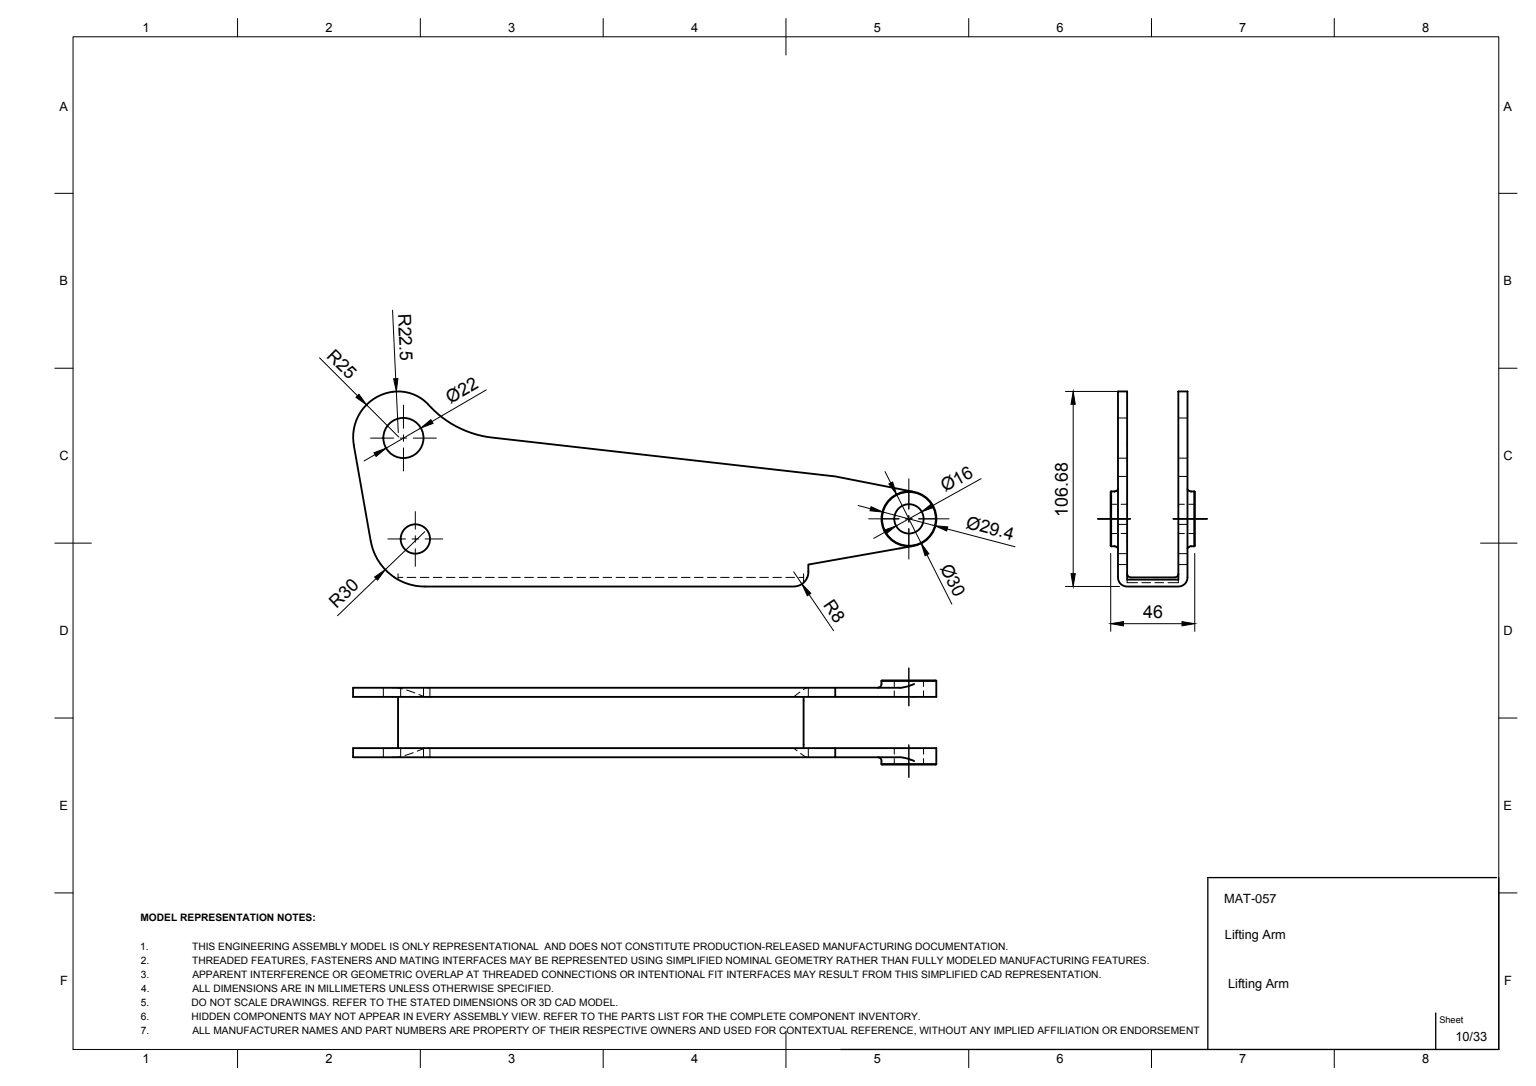
ISO-10303-21;
HEADER;
/* Generated by software containing ST-Developer
 * from STEP Tools, Inc. (www.steptools.com) 
 */

FILE_DESCRIPTION(
/* description */ ('STEP AP214', 'CAx-IF Rec.Pracs.---Representation and Presentation of Product Manufa
cturing Information (PMI)---4.0---2014-10-13'),
/* implementation_level */ '2;1');

FILE_NAME(
/* name */ 'Lifting Arm.step',
/* time_stamp */ '2026-10-28T23:34:22+01:00',
/* author */ (''),
/* organization */ (''),
/* preprocessor_version */ 'ST-DEVELOPER v20.2',
/* originating_system */ 'Autodesk Translation Framework v15.17.0.0',
/* authorisation */ '');

FILE_SCHEMA (('AP242_MANAGED_MODEL_BASED_3D_ENGINEERING_MIM_LF { 1 0 10303 442 2 1 4 }'));
ENDSEC;

DATA;
#10=MECHANICAL_DESIGN_GEOMETRIC_PRESENTATION_REPRESENTATION('',(#251),#27807);
#207=SHAPE_REPRESENTATION_RELATIONSHIP('SRR','None',#27902,#229);
#229=ADVANCED_BREP_SHAPE_REPRESENTATION('',(#280),#27782);
#251=STYLED_ITEM('',(#28070),#280);
#280=MANIFOLD_SOLID_BREP('Body1',#12027);
#363=FACE_BOUND('',#2137,.T.);
#364=FACE_BOUND('',#2138,.T.);
#365=FACE_BOUND('',#2142,.T.);
#366=FACE_BOUND('',#2143,.T.);
#367=FACE_BOUND('',#2144,.T.);
#368=FACE_BOUND('',#2152,.T.);
#369=FACE_BOUND('',#2153,.T.);
#370=FACE_BOUND('',#2178,.T.);
#371=FACE_BOUND('',#2179,.T.);
#372=FACE_BOUND('',#2180,.T.);
#373=FACE_BOUND('',#2182,.T.);
#374=FACE_BOUND('',#2184,.T.);
#514=PLANE('',#12657);
#515=PLANE('',#12665);
#516=PLANE('',#12669);
#517=PLANE('',#12678);
#518=PLANE('',#12681);
#519=PLANE('',#12684);
#520=PLANE('',#12685);
#521=PLANE('',#12686);
#522=PLANE('',#12693);
#523=PLANE('',#12721);
#524=PLANE('',#12726);
#525=PLANE('',#12727);
#526=PLANE('',#12728);
#527=PLANE('',#12729);
#528=PLANE('',#12730);
#529=PLANE('',#12731);
#530=PLANE('',#12732);
#531=PLANE('',#12733);
#532=PLANE('',#12735);
#533=PLANE('',#12736);
#534=PLANE('',#12739);
#535=PLANE('',#12742);
#825=TOROIDAL_SURFACE('',#12701,17.,2.);
#826=TOROIDAL_SURFACE('',#12704,17.,2.);
#866=B_SPLINE_CURVE_WITH_KNOTS('',3,(#18580,#18581,#18582,#18583,#18584,
#18585,#18586,#18587),.UNSPECIFIED.,.F.,.F.,(4,2,2,4),(1.64653183621645,
1.82629619953337,2.00606056285029,2.42476187739513),.UNSPECIFIED.);
#867=B_SPLINE_CURVE_WITH_KNOTS('',3,(#18614,#18615,#18616,#18617),
 .UNSPECIFIED.,.F.,.F.,(4,4),(0.,0.783684993176865),.UNSPECIFIED.);
#868=B_SPLINE_CURVE_WITH_KNOTS('',3,(#18636,#18637,#18638,#18639),
 .UNSPECIFIED.,.F.,.F.,(4,4),(-2.42476187739513,-1.64107688421826),
 .UNSPECIFIED.);
#869=B_SPLINE_CURVE_WITH_KNOTS('',3,(#18646,#18647,#18648,#18649,#18650,
#18651,#18652,#18653),.UNSPECIFIED.,.F.,.F.,(4,2,2,4),(-0.778230041178668,
-0.598465677861747,-0.418701314544826,0.),.UNSPECIFIED.);
#870=B_SPLINE_CURVE_WITH_KNOTS('',3,(#18695,#18696,#18697,#18698,#18699,
#18700,#18701,#18702),.UNSPECIFIED.,.F.,.F.,(4,2,2,4),(3.68263908945476,
4.12349601732247,4.56435294519017,5.44606680092558),.UNSPECIFIED.);
#871=B_SPLINE_CURVE_WITH_KNOTS('',3,(#18705,#18706,#18707,#18708,#18709,
#18710,#18711,#18712,#18713,#18714),.UNSPECIFIED.,.F.,.F.,(4,2,2,2,4),(0.,
0.473183086940068,0.946366173880136,1.33890283846488,1.73143950304963),
 .UNSPECIFIED.);
#872=B_SPLINE_CURVE_WITH_KNOTS('',3,(#18725,#18726,#18727,#18728,#18729,
#18730,#18731,#18732,#18733,#18734),.UNSPECIFIED.,.F.,.F.,(4,2,2,2,4),(0.,
0.287218434472245,0.57443686894449,0.807390418400316,1.04034396785614),
 .UNSPECIFIED.);
#873=B_SPLINE_CURVE_WITH_KNOTS('',3,(#18741,#18742,#18743,#18744,#18745,
#18746,#18747,#18748,#18749,#18750),.UNSPECIFIED.,.F.,.F.,(4,2,2,2,4),(2.56810417568796,
2.77815458546554,2.98820499524312,3.29809009872942,3.60797520221572),
 .UNSPECIFIED.);
#1048=CYLINDRICAL_SURFACE('',#12654,22.5);
#1049=CYLINDRICAL_SURFACE('',#12666,22.5);
#1050=CYLINDRICAL_SURFACE('',#12679,55.);
#1051=CYLINDRICAL_SURFACE('',#12682,55.);
#1052=CYLINDRICAL_SURFACE('',#12707,11.);
#1053=CYLINDRICAL_SURFACE('',#12708,7.99999999999999);
#1054=CYLINDRICAL_SURFACE('',#12709,7.99999999999999);
#1055=CYLINDRICAL_SURFACE('',#12711,15.);
#1056=CYLINDRICAL_SURFACE('',#12713,11.);
#1057=CYLINDRICAL_SURFACE('',#12715,7.99999999999999);
#1058=CYLINDRICAL_SURFACE('',#12717,7.99999999999999);
#1059=CYLINDRICAL_SURFACE('',#12720,15.);
#1060=CYLINDRICAL_SURFACE('',#12722,30.);
#1061=CYLINDRICAL_SURFACE('',#12724,7.99999999999999);
#1062=CYLINDRICAL_SURFACE('',#12737,25.);
#1063=CYLINDRICAL_SURFACE('',#12738,25.);
#1064=CYLINDRICAL_SURFACE('',#12745,5.);
#1065=CYLINDRICAL_SURFACE('',#12746,5.);
#1066=CYLINDRICAL_SURFACE('',#12747,2.);
#1067=CYLINDRICAL_SURFACE('',#12748,2.);
#1410=FACE_OUTER_BOUND('',#2135,.T.);
#1411=FACE_OUTER_BOUND('',#2136,.T.);
#1412=FACE_OUTER_BOUND('',#2139,.T.);
#1413=FACE_OUTER_BOUND('',#2140,.T.);
#1414=FACE_OUTER_BOUND('',#2141,.T.);
#1415=FACE_OUTER_BOUND('',#2145,.T.);
#1416=FACE_OUTER_BOUND('',#2146,.T.);
#1417=FACE_OUTER_BOUND('',#2147,.T.);
#1418=FACE_OUTER_BOUND('',#2148,.T.);
#1419=FACE_OUTER_BOUND('',#2149,.T.);
#1420=FACE_OUTER_BOUND('',#2150,.T.);
#1421=FACE_OUTER_BOUND('',#2151,.T.);
#1422=FACE_OUTER_BOUND('',#2154,.T.);
#1423=FACE_OUTER_BOUND('',#2155,.T.);
#1424=FACE_OUTER_BOUND('',#2156,.T.);
#1425=FACE_OUTER_BOUND('',#2157,.T.);
#1426=FACE_OUTER_BOUND('',#2158,.T.);
#1427=FACE_OUTER_BOUND('',#2159,.T.);
#1428=FACE_OUTER_BOUND('',#2160,.T.);
#1429=FACE_OUTER_BOUND('',#2161,.T.);
#1430=FACE_OUTER_BOUND('',#2162,.T.);
#1431=FACE_OUTER_BOUND('',#2163,.T.);
#1432=FACE_OUTER_BOUND('',#2164,.T.);
#1433=FACE_OUTER_BOUND('',#2165,.T.);
#1434=FACE_OUTER_BOUND('',#2166,.T.);
#1435=FACE_OUTER_BOUND('',#2167,.T.);
#1436=FACE_OUTER_BOUND('',#2168,.T.);
#1437=FACE_OUTER_BOUND('',#2169,.T.);
#1438=FACE_OUTER_BOUND('',#2170,.T.);
#1439=FACE_OUTER_BOUND('',#2171,.T.);
#1440=FACE_OUTER_BOUND('',#2172,.T.);
#1441=FACE_OUTER_BOUND('',#2173,.T.);
#1442=FACE_OUTER_BOUND('',#2174,.T.);
#1443=FACE_OUTER_BOUND('',#2175,.T.);
#1444=FACE_OUTER_BOUND('',#2176,.T.);
#1445=FACE_OUTER_BOUND('',#2177,.T.);
#1446=FACE_OUTER_BOUND('',#2181,.T.);
#1447=FACE_OUTER_BOUND('',#2183,.T.);
#1448=FACE_OUTER_BOUND('',#2185,.T.);
#1449=FACE_OUTER_BOUND('',#2186,.T.);
#1450=FACE_OUTER_BOUND('',#2187,.T.);
#1451=FACE_OUTER_BOUND('',#2188,.T.);
#1452=FACE_OUTER_BOUND('',#2189,.T.);
#1453=FACE_OUTER_BOUND('',#2190,.T.);
#1454=FACE_OUTER_BOUND('',#2191,.T.);
#1455=FACE_OUTER_BOUND('',#2192,.T.);
#2135=EDGE_LOOP('',(#8699,#8700,#8701,#8702));
#2136=EDGE_LOOP('',(#8703,#8704,#8705,#8706,#8707,#8708,#8709,#8710,#8711,
#8712,#8713,#8714,#8715));
#2137=EDGE_LOOP('',(#8716));
#2138=EDGE_LOOP('',(#8717));
#2139=EDGE_LOOP('',(#8718,#8719,#8720,#8721));
#2140=EDGE_LOOP('',(#8722,#8723,#8724,#8725));
#2141=EDGE_LOOP('',(#8726,#8727,#8728,#8729,#8730,#8731,#8732,#8733,#8734,
#8735,#8736,#8737,#8738,#8739,#8740));
#2142=EDGE_LOOP('',(#8741));
#2143=EDGE_LOOP('',(#8742));
#2144=EDGE_LOOP('',(#8743));
#2145=EDGE_LOOP('',(#8744,#8745,#8746,#8747));
#2146=EDGE_LOOP('',(#8748,#8749,#8750,#8751));
#2147=EDGE_LOOP('',(#8752,#8753,#8754,#8755));
#2148=EDGE_LOOP('',(#8756,#8757,#8758,#8759));
#2149=EDGE_LOOP('',(#8760,#8761,#8762,#8763));
#2150=EDGE_LOOP('',(#8764,#8765,#8766,#8767,#8768));
#2151=EDGE_LOOP('',(#8769,#8770,#8771,#8772,#8773,#8774,#8775,#8776,#8777,
#8778,#8779,#8780,#8781));
#2152=EDGE_LOOP('',(#8782));
#2153=EDGE_LOOP('',(#8783));
#2154=EDGE_LOOP('',(#8784,#8785,#8786,#8787,#8788));
#2155=EDGE_LOOP('',(#8789,#8790,#8791,#8792));
#2156=EDGE_LOOP('',(#8793,#8794,#8795,#8796,#8797));
#2157=EDGE_LOOP('',(#8798,#8799,#8800,#8801,#8802));
#2158=EDGE_LOOP('',(#8803,#8804,#8805,#8806,#8807));
#2159=EDGE_LOOP('',(#8808,#8809,#8810,#8811));
#2160=EDGE_LOOP('',(#8812,#8813,#8814,#8815));
#2161=EDGE_LOOP('',(#8816,#8817,#8818,#8819));
#2162=EDGE_LOOP('',(#8820,#8821,#8822,#8823,#8824,#8825,#8826,#8827,#8828));
#2163=EDGE_LOOP('',(#8829,#8830,#8831,#8832));
#2164=EDGE_LOOP('',(#8833,#8834,#8835,#8836));
#2165=EDGE_LOOP('',(#8837,#8838,#8839,#8840));
#2166=EDGE_LOOP('',(#8841,#8842,#8843,#8844,#8845,#8846,#8847,#8848));
#2167=EDGE_LOOP('',(#8849,#8850,#8851,#8852));
#2168=EDGE_LOOP('',(#8853,#8854,#8855,#8856,#8857,#8858,#8859,#8860,#8861,
#8862));
#2169=EDGE_LOOP('',(#8863,#8864,#8865,#8866,#8867,#8868,#8869,#8870,#8871,
#8872));
#2170=EDGE_LOOP('',(#8873,#8874,#8875,#8876));
#2171=EDGE_LOOP('',(#8877,#8878,#8879,#8880));
#2172=EDGE_LOOP('',(#8881,#8882,#8883,#8884,#8885));
#2173=EDGE_LOOP('',(#8886,#8887,#8888,#8889));
#2174=EDGE_LOOP('',(#8890,#8891,#8892,#8893));
#2175=EDGE_LOOP('',(#8894,#8895,#8896,#8897));
#2176=EDGE_LOOP('',(#8898,#8899,#8900,#8901,#8902));
#2177=EDGE_LOOP('',(#8903,#8904,#8905,#8906,#8907,#8908,#8909,#8910,#8911,
#8912,#8913,#8914,#8915,#8916,#8917));
#2178=EDGE_LOOP('',(#8918));
#2179=EDGE_LOOP('',(#8919));
#2180=EDGE_LOOP('',(#8920));
#2181=EDGE_LOOP('',(#8921));
#2182=EDGE_LOOP('',(#8922));
#2183=EDGE_LOOP('',(#8923));
#2184=EDGE_LOOP('',(#8924));
#2185=EDGE_LOOP('',(#8925,#8926,#8927,#8928));
#2186=EDGE_LOOP('',(#8929,#8930,#8931,#8932));
#2187=EDGE_LOOP('',(#8933,#8934,#8935,#8936,#8937,#8938));
#2188=EDGE_LOOP('',(#8939,#8940,#8941,#8942,#8943,#8944));
#2189=EDGE_LOOP('',(#8945,#8946,#8947,#8948));
#2190=EDGE_LOOP('',(#8949,#8950,#8951,#8952));
#2191=EDGE_LOOP('',(#8953,#8954,#8955,#8956));
#2192=EDGE_LOOP('',(#8957,#8958,#8959,#8960));
#2971=LINE('',#18477,#3791);
#2972=LINE('',#18480,#3792);
#2973=LINE('',#18483,#3793);
#2974=LINE('',#18487,#3794);
#2975=LINE('',#18489,#3795);
#2976=LINE('',#18493,#3796);
#2977=LINE('',#18495,#3797);
#2978=LINE('',#18499,#3798);
#2979=LINE('',#18503,#3799);
#2980=LINE('',#18511,#3800);
#2981=LINE('',#18512,#3801);
#2982=LINE('',#18518,#3802);
#2983=LINE('',#18521,#3803);
#2984=LINE('',#18524,#3804);
#2985=LINE('',#18528,#3805);
#2986=LINE('',#18530,#3806);
#2987=LINE('',#18534,#3807);
#2988=LINE('',#18536,#3808);
#2989=LINE('',#18540,#3809);
#2990=LINE('',#18542,#3810);
#2991=LINE('',#18544,#3811);
#2992=LINE('',#18548,#3812);
#2993=LINE('',#18558,#3813);
#2994=LINE('',#18559,#3814);
#2995=LINE('',#18563,#3815);
#2996=LINE('',#18566,#3816);
#2997=LINE('',#18567,#3817);
#2998=LINE('',#18571,#3818);
#2999=LINE('',#18574,#3819);
#3000=LINE('',#18575,#3820);
#3001=LINE('',#18578,#3821);
#3002=LINE('',#18588,#3822);
#3003=LINE('',#18593,#3823);
#3004=LINE('',#18597,#3824);
#3005=LINE('',#18601,#3825);
#3006=LINE('',#18603,#3826);
#3007=LINE('',#18611,#3827);
#3008=LINE('',#18613,#3828);
#3009=LINE('',#18622,#3829);
#3010=LINE('',#18630,#3830);
#3011=LINE('',#18655,#3831);
#3012=LINE('',#18657,#3832);
#3013=LINE('',#18661,#3833);
#3014=LINE('',#18663,#3834);
#3015=LINE('',#18666,#3835);
#3016=LINE('',#18670,#3836);
#3017=LINE('',#18674,#3837);
#3018=LINE('',#18679,#3838);
#3019=LINE('',#18682,#3839);
#3020=LINE('',#18683,#3840);
#3021=LINE('',#18687,#3841);
#3022=LINE('',#18689,#3842);
#3023=LINE('',#18691,#3843);
#3024=LINE('',#18692,#3844);
#3025=LINE('',#18704,#3845);
#3026=LINE('',#18715,#3846);
#3027=LINE('',#18717,#3847);
#3028=LINE('',#18720,#3848);
#3029=LINE('',#18724,#3849);
#3030=LINE('',#18736,#3850);
#3031=LINE('',#18739,#3851);
#3032=LINE('',#18740,#3852);
#3033=LINE('',#18752,#3853);
#3034=LINE('',#18755,#3854);
#3035=LINE('',#18756,#3855);
#3036=LINE('',#18759,#3856);
#3037=LINE('',#18760,#3857);
#3038=LINE('',#18762,#3858);
#3039=LINE('',#18764,#3859);
#3040=LINE('',#18765,#3860);
#3041=LINE('',#18767,#3861);
#3042=LINE('',#18772,#3862);
#3043=LINE('',#18774,#3863);
#3044=LINE('',#18775,#3864);
#3791=VECTOR('',#14665,22.5);
#3792=VECTOR('',#14668,22.5);
#3793=VECTOR('',#14671,10.);
#3794=VECTOR('',#14674,10.);
#3795=VECTOR('',#14675,1000.);
#3796=VECTOR('',#14678,1000.);
#3797=VECTOR('',#14679,1000.);
#3798=VECTOR('',#14682,1000.);
#3799=VECTOR('',#14685,1000.);
#3800=VECTOR('',#14694,10.);
#3801=VECTOR('',#14695,10.);
#3802=VECTOR('',#14700,22.5);
#3803=VECTOR('',#14703,22.5);
#3804=VECTOR('',#14706,10.);
#3805=VECTOR('',#14709,10.);
#3806=VECTOR('',#14710,1000.);
#3807=VECTOR('',#14713,1000.);
#3808=VECTOR('',#14714,1000.);
#3809=VECTOR('',#14717,1000.);
#3810=VECTOR('',#14718,1000.);
#3811=VECTOR('',#14719,1000.);
#3812=VECTOR('',#14722,1000.);
#3813=VECTOR('',#14733,10.);
#3814=VECTOR('',#14734,10.);
#3815=VECTOR('',#14739,10.);
#3816=VECTOR('',#14742,10.);
#3817=VECTOR('',#14743,10.);
#3818=VECTOR('',#14748,10.);
#3819=VECTOR('',#14751,10.);
#3820=VECTOR('',#14752,10.);
#3821=VECTOR('',#14755,1000.);
#3822=VECTOR('',#14756,1000.);
#3823=VECTOR('',#14761,1000.);
#3824=VECTOR('',#14764,1000.);
#3825=VECTOR('',#14767,1000.);
#3826=VECTOR('',#14768,1000.);
#3827=VECTOR('',#14777,1000.);
#3828=VECTOR('',#14778,1000.);
#3829=VECTOR('',#14783,14.7);
#3830=VECTOR('',#14792,15.);
#3831=VECTOR('',#14809,11.);
#3832=VECTOR('',#14812,7.99999999999999);
#3833=VECTOR('',#14817,7.99999999999999);
#3834=VECTOR('',#14820,15.);
#3835=VECTOR('',#14823,1000.);
#3836=VECTOR('',#14828,11.);
#3837=VECTOR('',#14833,7.99999999999999);
#3838=VECTOR('',#14838,7.99999999999999);
#3839=VECTOR('',#14843,15.);
#3840=VECTOR('',#14844,1000.);
#3841=VECTOR('',#14847,1000.);
#3842=VECTOR('',#14848,1000.);
#3843=VECTOR('',#14849,1000.);
#3844=VECTOR('',#14850,1000.);
#3845=VECTOR('',#14853,1000.);
#3846=VECTOR('',#14854,1000.);
#3847=VECTOR('',#14855,1000.);
#3848=VECTOR('',#14858,1000.);
#3849=VECTOR('',#14861,1000.);
#3850=VECTOR('',#14862,1000.);
#3851=VECTOR('',#14865,1000.);
#3852=VECTOR('',#14866,1000.);
#3853=VECTOR('',#14869,1000.);
#3854=VECTOR('',#14872,1000.);
#3855=VECTOR('',#14873,1000.);
#3856=VECTOR('',#14876,1000.);
#3857=VECTOR('',#14877,1000.);
#3858=VECTOR('',#14880,1000.);
#3859=VECTOR('',#14883,1000.);
#3860=VECTOR('',#14884,1000.);
#3861=VECTOR('',#14887,1000.);
#3862=VECTOR('',#14894,1000.);
#3863=VECTOR('',#14895,1000.);
#3864=VECTOR('',#14896,1000.);
#4560=CIRCLE('',#12655,22.5);
#4561=CIRCLE('',#12656,22.5);
#4562=CIRCLE('',#12658,55.);
#4563=CIRCLE('',#12659,17.);
#4564=CIRCLE('',#12660,7.99999999999999);
#4565=CIRCLE('',#12661,30.);
#4566=CIRCLE('',#12662,25.);
#4567=CIRCLE('',#12663,7.99999999999999);
#4568=CIRCLE('',#12664,11.);
#4569=CIRCLE('',#12667,22.5);
#4570=CIRCLE('',#12668,22.5);
#4571=CIRCLE('',#12670,55.);
#4572=CIRCLE('',#12671,15.);
#4573=CIRCLE('',#12672,7.99999999999999);
#4574=CIRCLE('',#12673,30.);
#4575=CIRCLE('',#12674,25.);
#4576=CIRCLE('',#12675,11.);
#4577=CIRCLE('',#12676,7.99999999999999);
#4578=CIRCLE('',#12677,7.99999999999999);
#4579=CIRCLE('',#12680,55.);
#4580=CIRCLE('',#12683,55.);
#4581=CIRCLE('',#12687,25.);
#4582=CIRCLE('',#12688,30.);
#4583=CIRCLE('',#12689,7.99999999999999);
#4584=CIRCLE('',#12690,17.);
#4585=CIRCLE('',#12691,11.);
#4586=CIRCLE('',#12692,7.99999999999999);
#4587=CIRCLE('',#12695,15.);
#4588=CIRCLE('',#12696,14.7);
#4589=CIRCLE('',#12698,15.);
#4590=CIRCLE('',#12699,15.);
#4591=CIRCLE('',#12700,14.7);
#4592=CIRCLE('',#12702,15.);
#4593=CIRCLE('',#12703,15.);
#4594=CIRCLE('',#12705,15.);
#4595=CIRCLE('',#12706,15.);
#4596=CIRCLE('',#12710,7.99999999999999);
#4597=CIRCLE('',#12712,15.);
#4598=CIRCLE('',#12714,11.);
#4599=CIRCLE('',#12716,7.99999999999999);
#4600=CIRCLE('',#12718,7.99999999999999);
#4601=CIRCLE('',#12719,7.99999999999999);
#4602=CIRCLE('',#12723,30.);
#4603=CIRCLE('',#12725,7.99999999999999);
#4604=CIRCLE('',#12734,25.);
#4605=CIRCLE('',#12740,2.);
#4606=CIRCLE('',#12741,2.);
#4607=CIRCLE('',#12743,2.);
#4608=CIRCLE('',#12744,2.);
#5306=VERTEX_POINT('',#18473);
#5307=VERTEX_POINT('',#18474);
#5308=VERTEX_POINT('',#18476);
#5309=VERTEX_POINT('',#18478);
#5310=VERTEX_POINT('',#18482);
#5311=VERTEX_POINT('',#18484);
#5312=VERTEX_POINT('',#18486);
#5313=VERTEX_POINT('',#18488);
#5314=VERTEX_POINT('',#18490);
#5315=VERTEX_POINT('',#18492);
#5316=VERTEX_POINT('',#18494);
#5317=VERTEX_POINT('',#18496);
#5318=VERTEX_POINT('',#18498);
#5319=VERTEX_POINT('',#18500);
#5320=VERTEX_POINT('',#18502);
#5321=VERTEX_POINT('',#18505);
#5322=VERTEX_POINT('',#18507);
#5323=VERTEX_POINT('',#18510);
#5324=VERTEX_POINT('',#18514);
#5325=VERTEX_POINT('',#18515);
#5326=VERTEX_POINT('',#18517);
#5327=VERTEX_POINT('',#18519);
#5328=VERTEX_POINT('',#18523);
#5329=VERTEX_POINT('',#18525);
#5330=VERTEX_POINT('',#18527);
#5331=VERTEX_POINT('',#18529);
#5332=VERTEX_POINT('',#18531);
#5333=VERTEX_POINT('',#18533);
#5334=VERTEX_POINT('',#18535);
#5335=VERTEX_POINT('',#18537);
#5336=VERTEX_POINT('',#18539);
#5337=VERTEX_POINT('',#18541);
#5338=VERTEX_POINT('',#18543);
#5339=VERTEX_POINT('',#18545);
#5340=VERTEX_POINT('',#18547);
#5341=VERTEX_POINT('',#18550);
#5342=VERTEX_POINT('',#18552);
#5343=VERTEX_POINT('',#18554);
#5344=VERTEX_POINT('',#18557);
#5345=VERTEX_POINT('',#18561);
#5346=VERTEX_POINT('',#18565);
#5347=VERTEX_POINT('',#18569);
#5348=VERTEX_POINT('',#18573);
#5349=VERTEX_POINT('',#18577);
#5350=VERTEX_POINT('',#18579);
#5351=VERTEX_POINT('',#18590);
#5352=VERTEX_POINT('',#18592);
#5353=VERTEX_POINT('',#18594);
#5354=VERTEX_POINT('',#18596);
#5355=VERTEX_POINT('',#18598);
#5356=VERTEX_POINT('',#18600);
#5357=VERTEX_POINT('',#18602);
#5358=VERTEX_POINT('',#18605);
#5359=VERTEX_POINT('',#18607);
#5360=VERTEX_POINT('',#18610);
#5361=VERTEX_POINT('',#18612);
#5362=VERTEX_POINT('',#18619);
#5363=VERTEX_POINT('',#18621);
#5364=VERTEX_POINT('',#18625);
#5365=VERTEX_POINT('',#18626);
#5366=VERTEX_POINT('',#18629);
#5367=VERTEX_POINT('',#18633);
#5368=VERTEX_POINT('',#18635);
#5369=VERTEX_POINT('',#18642);
#5370=VERTEX_POINT('',#18644);
#5371=VERTEX_POINT('',#18659);
#5372=VERTEX_POINT('',#18664);
#5373=VERTEX_POINT('',#18668);
#5374=VERTEX_POINT('',#18672);
#5375=VERTEX_POINT('',#18676);
#5376=VERTEX_POINT('',#18678);
#5377=VERTEX_POINT('',#18685);
#5378=VERTEX_POINT('',#18686);
#5379=VERTEX_POINT('',#18688);
#5380=VERTEX_POINT('',#18690);
#5381=VERTEX_POINT('',#18694);
#5382=VERTEX_POINT('',#18703);
#5383=VERTEX_POINT('',#18716);
#5384=VERTEX_POINT('',#18718);
#5385=VERTEX_POINT('',#18722);
#5386=VERTEX_POINT('',#18723);
#5387=VERTEX_POINT('',#18735);
#5388=VERTEX_POINT('',#18737);
#5389=VERTEX_POINT('',#18754);
#5390=VERTEX_POINT('',#18758);
#5391=VERTEX_POINT('',#18771);
#5392=VERTEX_POINT('',#18773);
#6562=EDGE_CURVE('',#5306,#5307,#4560,.T.);
#6563=EDGE_CURVE('',#5307,#5308,#2971,.T.);
#6564=EDGE_CURVE('',#5308,#5309,#4561,.T.);
#6565=EDGE_CURVE('',#5309,#5306,#2972,.T.);
#6566=EDGE_CURVE('',#5306,#5310,#2973,.T.);
#6567=EDGE_CURVE('',#5311,#5310,#4562,.T.);
#6568=EDGE_CURVE('',#5311,#5312,#2974,.T.);
#6569=EDGE_CURVE('',#5313,#5312,#2975,.T.);
#6570=EDGE_CURVE('',#5313,#5314,#4563,.T.);
#6571=EDGE_CURVE('',#5315,#5314,#2976,.T.);
#6572=EDGE_CURVE('',#5316,#5315,#2977,.T.);
#6573=EDGE_CURVE('',#5316,#5317,#4564,.T.);
#6574=EDGE_CURVE('',#5317,#5318,#2978,.T.);
#6575=EDGE_CURVE('',#5318,#5319,#4565,.T.);
#6576=EDGE_CURVE('',#5320,#5319,#2979,.T.);
#6577=EDGE_CURVE('',#5320,#5307,#4566,.T.);
#6578=EDGE_CURVE('',#5321,#5321,#4567,.T.);
#6579=EDGE_CURVE('',#5322,#5322,#4568,.T.);
#6580=EDGE_CURVE('',#5323,#5309,#2980,.T.);
#6581=EDGE_CURVE('',#5310,#5323,#2981,.T.);
#6582=EDGE_CURVE('',#5324,#5325,#4569,.T.);
#6583=EDGE_CURVE('',#5325,#5326,#2982,.T.);
#6584=EDGE_CURVE('',#5326,#5327,#4570,.T.);
#6585=EDGE_CURVE('',#5327,#5324,#2983,.T.);
#6586=EDGE_CURVE('',#5324,#5328,#2984,.T.);
#6587=EDGE_CURVE('',#5329,#5328,#4571,.T.);
#6588=EDGE_CURVE('',#5329,#5330,#2985,.T.);
#6589=EDGE_CURVE('',#5331,#5330,#2986,.T.);
#6590=EDGE_CURVE('',#5332,#5331,#4572,.T.);
#6591=EDGE_CURVE('',#5333,#5332,#2987,.T.);
#6592=EDGE_CURVE('',#5334,#5333,#2988,.T.);
#6593=EDGE_CURVE('',#5334,#5335,#4573,.T.);
#6594=EDGE_CURVE('',#5336,#5335,#2989,.T.);
#6595=EDGE_CURVE('',#5336,#5337,#2990,.T.);
#6596=EDGE_CURVE('',#5337,#5338,#2991,.T.);
#6597=EDGE_CURVE('',#5338,#5339,#4574,.T.);
#6598=EDGE_CURVE('',#5340,#5339,#2992,.T.);
#6599=EDGE_CURVE('',#5340,#5325,#4575,.T.);
#6600=EDGE_CURVE('',#5341,#5341,#4576,.T.);
#6601=EDGE_CURVE('',#5342,#5342,#4577,.T.);
#6602=EDGE_CURVE('',#5343,#5343,#4578,.T.);
#6603=EDGE_CURVE('',#5344,#5327,#2993,.T.);
#6604=EDGE_CURVE('',#5328,#5344,#2994,.T.);
#6605=EDGE_CURVE('',#5323,#5345,#4579,.T.);
#6606=EDGE_CURVE('',#5345,#5311,#2995,.T.);
#6607=EDGE_CURVE('',#5346,#5345,#2996,.T.);
#6608=EDGE_CURVE('',#5312,#5346,#2997,.T.);
#6609=EDGE_CURVE('',#5344,#5347,#4580,.T.);
#6610=EDGE_CURVE('',#5347,#5329,#2998,.T.);
#6611=EDGE_CURVE('',#5348,#5347,#2999,.T.);
#6612=EDGE_CURVE('',#5330,#5348,#3000,.T.);
#6613=EDGE_CURVE('',#5349,#5348,#3001,.T.);
#6614=EDGE_CURVE('',#5349,#5350,#866,.T.);
#6615=EDGE_CURVE('',#5350,#5331,#3002,.T.);
#6616=EDGE_CURVE('',#5326,#5351,#4581,.T.);
#6617=EDGE_CURVE('',#5351,#5352,#3003,.T.);
#6618=EDGE_CURVE('',#5352,#5353,#4582,.T.);
#6619=EDGE_CURVE('',#5353,#5354,#3004,.T.);
#6620=EDGE_CURVE('',#5354,#5355,#4583,.T.);
#6621=EDGE_CURVE('',#5355,#5356,#3005,.T.);
#6622=EDGE_CURVE('',#5356,#5357,#3006,.T.);
#6623=EDGE_CURVE('',#5357,#5349,#4584,.T.);
#6624=EDGE_CURVE('',#5358,#5358,#4585,.T.);
#6625=EDGE_CURVE('',#5359,#5359,#4586,.T.);
#6626=EDGE_CURVE('',#5346,#5360,#3007,.T.);
#6627=EDGE_CURVE('',#5360,#5361,#3008,.T.);
#6628=EDGE_CURVE('',#5361,#5313,#867,.T.);
#6629=EDGE_CURVE('',#5362,#5362,#4587,.T.);
#6630=EDGE_CURVE('',#5362,#5363,#3009,.T.);
#6631=EDGE_CURVE('',#5363,#5363,#4588,.T.);
#6632=EDGE_CURVE('',#5364,#5365,#4589,.T.);
#6633=EDGE_CURVE('',#5365,#5364,#4590,.T.);
#6634=EDGE_CURVE('',#5365,#5366,#3010,.T.);
#6635=EDGE_CURVE('',#5366,#5366,#4591,.T.);
#6636=EDGE_CURVE('',#5350,#5367,#4592,.T.);
#6637=EDGE_CURVE('',#5368,#5357,#868,.T.);
#6638=EDGE_CURVE('',#5367,#5368,#4593,.T.);
#6639=EDGE_CURVE('',#5369,#5361,#4594,.T.);
#6640=EDGE_CURVE('',#5370,#5369,#4595,.T.);
#6641=EDGE_CURVE('',#5314,#5370,#869,.T.);
#6642=EDGE_CURVE('',#5358,#5341,#3011,.T.);
#6643=EDGE_CURVE('',#5359,#5343,#3012,.T.);
#6644=EDGE_CURVE('',#5371,#5371,#4596,.T.);
#6645=EDGE_CURVE('',#5371,#5342,#3013,.T.);
#6646=EDGE_CURVE('',#5364,#5369,#3014,.T.);
#6647=EDGE_CURVE('',#5360,#5372,#4597,.T.);
#6648=EDGE_CURVE('',#5372,#5370,#3015,.T.);
#6649=EDGE_CURVE('',#5373,#5373,#4598,.T.);
#6650=EDGE_CURVE('',#5373,#5322,#3016,.T.);
#6651=EDGE_CURVE('',#5374,#5374,#4599,.T.);
#6652=EDGE_CURVE('',#5374,#5321,#3017,.T.);
#6653=EDGE_CURVE('',#5375,#5375,#4600,.T.);
#6654=EDGE_CURVE('',#5375,#5376,#3018,.T.);
#6655=EDGE_CURVE('',#5376,#5376,#4601,.T.);
#6656=EDGE_CURVE('',#5367,#5362,#3019,.T.);
#6657=EDGE_CURVE('',#5368,#5332,#3020,.T.);
#6658=EDGE_CURVE('',#5377,#5378,#3021,.T.);
#6659=EDGE_CURVE('',#5377,#5379,#3022,.T.);
#6660=EDGE_CURVE('',#5380,#5379,#3023,.T.);
#6661=EDGE_CURVE('',#5380,#5378,#3024,.T.);
#6662=EDGE_CURVE('',#5318,#5381,#870,.T.);
#6663=EDGE_CURVE('',#5382,#5381,#3025,.T.);
#6664=EDGE_CURVE('',#5382,#5353,#871,.T.);
#6665=EDGE_CURVE('',#5339,#5352,#3026,.T.);
#6666=EDGE_CURVE('',#5338,#5383,#3027,.T.);
#6667=EDGE_CURVE('',#5384,#5383,#4602,.T.);
#6668=EDGE_CURVE('',#5319,#5384,#3028,.T.);
#6669=EDGE_CURVE('',#5385,#5386,#3029,.T.);
#6670=EDGE_CURVE('',#5385,#5317,#872,.T.);
#6671=EDGE_CURVE('',#5387,#5316,#3030,.T.);
#6672=EDGE_CURVE('',#5388,#5387,#4603,.T.);
#6673=EDGE_CURVE('',#5388,#5335,#3031,.T.);
#6674=EDGE_CURVE('',#5355,#5334,#3032,.T.);
#6675=EDGE_CURVE('',#5354,#5386,#873,.T.);
#6676=EDGE_CURVE('',#5356,#5333,#3033,.T.);
#6677=EDGE_CURVE('',#5384,#5389,#3034,.T.);
#6678=EDGE_CURVE('',#5389,#5320,#3035,.T.);
#6679=EDGE_CURVE('',#5372,#5390,#3036,.T.);
#6680=EDGE_CURVE('',#5390,#5315,#3037,.T.);
#6681=EDGE_CURVE('',#5351,#5340,#3038,.T.);
#6682=EDGE_CURVE('',#5381,#5385,#3039,.T.);
#6683=EDGE_CURVE('',#5386,#5382,#3040,.T.);
#6684=EDGE_CURVE('',#5390,#5387,#3041,.T.);
#6685=EDGE_CURVE('',#5308,#5389,#4604,.T.);
#6686=EDGE_CURVE('',#5391,#5383,#3042,.T.);
#6687=EDGE_CURVE('',#5391,#5392,#3043,.T.);
#6688=EDGE_CURVE('',#5392,#5388,#3044,.T.);
#6689=EDGE_CURVE('',#5392,#5377,#4605,.T.);
#6690=EDGE_CURVE('',#5378,#5336,#4606,.T.);
#6691=EDGE_CURVE('',#5337,#5380,#4607,.T.);
#6692=EDGE_CURVE('',#5379,#5391,#4608,.T.);
#8699=ORIENTED_EDGE('',*,*,#6562,.T.);
#8700=ORIENTED_EDGE('',*,*,#6563,.T.);
#8701=ORIENTED_EDGE('',*,*,#6564,.T.);
#8702=ORIENTED_EDGE('',*,*,#6565,.T.);
#8703=ORIENTED_EDGE('',*,*,#6562,.F.);
#8704=ORIENTED_EDGE('',*,*,#6566,.T.);
#8705=ORIENTED_EDGE('',*,*,#6567,.F.);
#8706=ORIENTED_EDGE('',*,*,#6568,.T.);
#8707=ORIENTED_EDGE('',*,*,#6569,.F.);
#8708=ORIENTED_EDGE('',*,*,#6570,.T.);
#8709=ORIENTED_EDGE('',*,*,#6571,.F.);
#8710=ORIENTED_EDGE('',*,*,#6572,.F.);
#8711=ORIENTED_EDGE('',*,*,#6573,.T.);
#8712=ORIENTED_EDGE('',*,*,#6574,.T.);
#8713=ORIENTED_EDGE('',*,*,#6575,.T.);
#8714=ORIENTED_EDGE('',*,*,#6576,.F.);
#8715=ORIENTED_EDGE('',*,*,#6577,.T.);
#8716=ORIENTED_EDGE('',*,*,#6578,.T.);
#8717=ORIENTED_EDGE('',*,*,#6579,.T.);
#8718=ORIENTED_EDGE('',*,*,#6565,.F.);
#8719=ORIENTED_EDGE('',*,*,#6580,.F.);
#8720=ORIENTED_EDGE('',*,*,#6581,.F.);
#8721=ORIENTED_EDGE('',*,*,#6566,.F.);
#8722=ORIENTED_EDGE('',*,*,#6582,.T.);
#8723=ORIENTED_EDGE('',*,*,#6583,.T.);
#8724=ORIENTED_EDGE('',*,*,#6584,.T.);
#8725=ORIENTED_EDGE('',*,*,#6585,.T.);
#8726=ORIENTED_EDGE('',*,*,#6582,.F.);
#8727=ORIENTED_EDGE('',*,*,#6586,.T.);
#8728=ORIENTED_EDGE('',*,*,#6587,.F.);
#8729=ORIENTED_EDGE('',*,*,#6588,.T.);
#8730=ORIENTED_EDGE('',*,*,#6589,.F.);
#8731=ORIENTED_EDGE('',*,*,#6590,.F.);
#8732=ORIENTED_EDGE('',*,*,#6591,.F.);
#8733=ORIENTED_EDGE('',*,*,#6592,.F.);
#8734=ORIENTED_EDGE('',*,*,#6593,.T.);
#8735=ORIENTED_EDGE('',*,*,#6594,.F.);
#8736=ORIENTED_EDGE('',*,*,#6595,.T.);
#8737=ORIENTED_EDGE('',*,*,#6596,.T.);
#8738=ORIENTED_EDGE('',*,*,#6597,.T.);
#8739=ORIENTED_EDGE('',*,*,#6598,.F.);
#8740=ORIENTED_EDGE('',*,*,#6599,.T.);
#8741=ORIENTED_EDGE('',*,*,#6600,.T.);
#8742=ORIENTED_EDGE('',*,*,#6601,.T.);
#8743=ORIENTED_EDGE('',*,*,#6602,.T.);
#8744=ORIENTED_EDGE('',*,*,#6585,.F.);
#8745=ORIENTED_EDGE('',*,*,#6603,.F.);
#8746=ORIENTED_EDGE('',*,*,#6604,.F.);
#8747=ORIENTED_EDGE('',*,*,#6586,.F.);
#8748=ORIENTED_EDGE('',*,*,#6605,.T.);
#8749=ORIENTED_EDGE('',*,*,#6606,.T.);
#8750=ORIENTED_EDGE('',*,*,#6567,.T.);
#8751=ORIENTED_EDGE('',*,*,#6581,.T.);
#8752=ORIENTED_EDGE('',*,*,#6606,.F.);
#8753=ORIENTED_EDGE('',*,*,#6607,.F.);
#8754=ORIENTED_EDGE('',*,*,#6608,.F.);
#8755=ORIENTED_EDGE('',*,*,#6568,.F.);
#8756=ORIENTED_EDGE('',*,*,#6609,.T.);
#8757=ORIENTED_EDGE('',*,*,#6610,.T.);
#8758=ORIENTED_EDGE('',*,*,#6587,.T.);
#8759=ORIENTED_EDGE('',*,*,#6604,.T.);
#8760=ORIENTED_EDGE('',*,*,#6610,.F.);
#8761=ORIENTED_EDGE('',*,*,#6611,.F.);
#8762=ORIENTED_EDGE('',*,*,#6612,.F.);
#8763=ORIENTED_EDGE('',*,*,#6588,.F.);
#8764=ORIENTED_EDGE('',*,*,#6612,.T.);
#8765=ORIENTED_EDGE('',*,*,#6613,.F.);
#8766=ORIENTED_EDGE('',*,*,#6614,.T.);
#8767=ORIENTED_EDGE('',*,*,#6615,.T.);
#8768=ORIENTED_EDGE('',*,*,#6589,.T.);
#8769=ORIENTED_EDGE('',*,*,#6584,.F.);
#8770=ORIENTED_EDGE('',*,*,#6616,.T.);
#8771=ORIENTED_EDGE('',*,*,#6617,.T.);
#8772=ORIENTED_EDGE('',*,*,#6618,.T.);
#8773=ORIENTED_EDGE('',*,*,#6619,.T.);
#8774=ORIENTED_EDGE('',*,*,#6620,.T.);
#8775=ORIENTED_EDGE('',*,*,#6621,.T.);
#8776=ORIENTED_EDGE('',*,*,#6622,.T.);
#8777=ORIENTED_EDGE('',*,*,#6623,.T.);
#8778=ORIENTED_EDGE('',*,*,#6613,.T.);
#8779=ORIENTED_EDGE('',*,*,#6611,.T.);
#8780=ORIENTED_EDGE('',*,*,#6609,.F.);
#8781=ORIENTED_EDGE('',*,*,#6603,.T.);
#8782=ORIENTED_EDGE('',*,*,#6624,.F.);
#8783=ORIENTED_EDGE('',*,*,#6625,.F.);
#8784=ORIENTED_EDGE('',*,*,#6608,.T.);
#8785=ORIENTED_EDGE('',*,*,#6626,.T.);
#8786=ORIENTED_EDGE('',*,*,#6627,.T.);
#8787=ORIENTED_EDGE('',*,*,#6628,.T.);
#8788=ORIENTED_EDGE('',*,*,#6569,.T.);
#8789=ORIENTED_EDGE('',*,*,#6629,.F.);
#8790=ORIENTED_EDGE('',*,*,#6630,.T.);
#8791=ORIENTED_EDGE('',*,*,#6631,.F.);
#8792=ORIENTED_EDGE('',*,*,#6630,.F.);
#8793=ORIENTED_EDGE('',*,*,#6632,.F.);
#8794=ORIENTED_EDGE('',*,*,#6633,.F.);
#8795=ORIENTED_EDGE('',*,*,#6634,.T.);
#8796=ORIENTED_EDGE('',*,*,#6635,.F.);
#8797=ORIENTED_EDGE('',*,*,#6634,.F.);
#8798=ORIENTED_EDGE('',*,*,#6636,.F.);
#8799=ORIENTED_EDGE('',*,*,#6614,.F.);
#8800=ORIENTED_EDGE('',*,*,#6623,.F.);
#8801=ORIENTED_EDGE('',*,*,#6637,.F.);
#8802=ORIENTED_EDGE('',*,*,#6638,.F.);
#8803=ORIENTED_EDGE('',*,*,#6570,.F.);
#8804=ORIENTED_EDGE('',*,*,#6628,.F.);
#8805=ORIENTED_EDGE('',*,*,#6639,.F.);
#8806=ORIENTED_EDGE('',*,*,#6640,.F.);
#8807=ORIENTED_EDGE('',*,*,#6641,.F.);
#8808=ORIENTED_EDGE('',*,*,#6624,.T.);
#8809=ORIENTED_EDGE('',*,*,#6642,.T.);
#8810=ORIENTED_EDGE('',*,*,#6600,.F.);
#8811=ORIENTED_EDGE('',*,*,#6642,.F.);
#8812=ORIENTED_EDGE('',*,*,#6625,.T.);
#8813=ORIENTED_EDGE('',*,*,#6643,.T.);
#8814=ORIENTED_EDGE('',*,*,#6602,.F.);
#8815=ORIENTED_EDGE('',*,*,#6643,.F.);
#8816=ORIENTED_EDGE('',*,*,#6644,.T.);
#8817=ORIENTED_EDGE('',*,*,#6645,.T.);
#8818=ORIENTED_EDGE('',*,*,#6601,.F.);
#8819=ORIENTED_EDGE('',*,*,#6645,.F.);
#8820=ORIENTED_EDGE('',*,*,#6632,.T.);
#8821=ORIENTED_EDGE('',*,*,#6633,.T.);
#8822=ORIENTED_EDGE('',*,*,#6646,.T.);
#8823=ORIENTED_EDGE('',*,*,#6639,.T.);
#8824=ORIENTED_EDGE('',*,*,#6627,.F.);
#8825=ORIENTED_EDGE('',*,*,#6647,.T.);
#8826=ORIENTED_EDGE('',*,*,#6648,.T.);
#8827=ORIENTED_EDGE('',*,*,#6640,.T.);
#8828=ORIENTED_EDGE('',*,*,#6646,.F.);
#8829=ORIENTED_EDGE('',*,*,#6649,.F.);
#8830=ORIENTED_EDGE('',*,*,#6650,.T.);
#8831=ORIENTED_EDGE('',*,*,#6579,.F.);
#8832=ORIENTED_EDGE('',*,*,#6650,.F.);
#8833=ORIENTED_EDGE('',*,*,#6651,.F.);
#8834=ORIENTED_EDGE('',*,*,#6652,.T.);
#8835=ORIENTED_EDGE('',*,*,#6578,.F.);
#8836=ORIENTED_EDGE('',*,*,#6652,.F.);
#8837=ORIENTED_EDGE('',*,*,#6653,.F.);
#8838=ORIENTED_EDGE('',*,*,#6654,.T.);
#8839=ORIENTED_EDGE('',*,*,#6655,.F.);
#8840=ORIENTED_EDGE('',*,*,#6654,.F.);
#8841=ORIENTED_EDGE('',*,*,#6590,.T.);
#8842=ORIENTED_EDGE('',*,*,#6615,.F.);
#8843=ORIENTED_EDGE('',*,*,#6636,.T.);
#8844=ORIENTED_EDGE('',*,*,#6656,.T.);
#8845=ORIENTED_EDGE('',*,*,#6629,.T.);
#8846=ORIENTED_EDGE('',*,*,#6656,.F.);
#8847=ORIENTED_EDGE('',*,*,#6638,.T.);
#8848=ORIENTED_EDGE('',*,*,#6657,.T.);
#8849=ORIENTED_EDGE('',*,*,#6658,.F.);
#8850=ORIENTED_EDGE('',*,*,#6659,.T.);
#8851=ORIENTED_EDGE('',*,*,#6660,.F.);
#8852=ORIENTED_EDGE('',*,*,#6661,.T.);
#8853=ORIENTED_EDGE('',*,*,#6575,.F.);
#8854=ORIENTED_EDGE('',*,*,#6662,.T.);
#8855=ORIENTED_EDGE('',*,*,#6663,.F.);
#8856=ORIENTED_EDGE('',*,*,#6664,.T.);
#8857=ORIENTED_EDGE('',*,*,#6618,.F.);
#8858=ORIENTED_EDGE('',*,*,#6665,.F.);
#8859=ORIENTED_EDGE('',*,*,#6597,.F.);
#8860=ORIENTED_EDGE('',*,*,#6666,.T.);
#8861=ORIENTED_EDGE('',*,*,#6667,.F.);
#8862=ORIENTED_EDGE('',*,*,#6668,.F.);
#8863=ORIENTED_EDGE('',*,*,#6669,.F.);
#8864=ORIENTED_EDGE('',*,*,#6670,.T.);
#8865=ORIENTED_EDGE('',*,*,#6573,.F.);
#8866=ORIENTED_EDGE('',*,*,#6671,.F.);
#8867=ORIENTED_EDGE('',*,*,#6672,.F.);
#8868=ORIENTED_EDGE('',*,*,#6673,.T.);
#8869=ORIENTED_EDGE('',*,*,#6593,.F.);
#8870=ORIENTED_EDGE('',*,*,#6674,.F.);
#8871=ORIENTED_EDGE('',*,*,#6620,.F.);
#8872=ORIENTED_EDGE('',*,*,#6675,.T.);
#8873=ORIENTED_EDGE('',*,*,#6621,.F.);
#8874=ORIENTED_EDGE('',*,*,#6674,.T.);
#8875=ORIENTED_EDGE('',*,*,#6592,.T.);
#8876=ORIENTED_EDGE('',*,*,#6676,.F.);
#8877=ORIENTED_EDGE('',*,*,#6677,.T.);
#8878=ORIENTED_EDGE('',*,*,#6678,.T.);
#8879=ORIENTED_EDGE('',*,*,#6576,.T.);
#8880=ORIENTED_EDGE('',*,*,#6668,.T.);
#8881=ORIENTED_EDGE('',*,*,#6648,.F.);
#8882=ORIENTED_EDGE('',*,*,#6679,.T.);
#8883=ORIENTED_EDGE('',*,*,#6680,.T.);
#8884=ORIENTED_EDGE('',*,*,#6571,.T.);
#8885=ORIENTED_EDGE('',*,*,#6641,.T.);
#8886=ORIENTED_EDGE('',*,*,#6617,.F.);
#8887=ORIENTED_EDGE('',*,*,#6681,.T.);
#8888=ORIENTED_EDGE('',*,*,#6598,.T.);
#8889=ORIENTED_EDGE('',*,*,#6665,.T.);
#8890=ORIENTED_EDGE('',*,*,#6663,.T.);
#8891=ORIENTED_EDGE('',*,*,#6682,.T.);
#8892=ORIENTED_EDGE('',*,*,#6669,.T.);
#8893=ORIENTED_EDGE('',*,*,#6683,.T.);
#8894=ORIENTED_EDGE('',*,*,#6684,.T.);
#8895=ORIENTED_EDGE('',*,*,#6671,.T.);
#8896=ORIENTED_EDGE('',*,*,#6572,.T.);
#8897=ORIENTED_EDGE('',*,*,#6680,.F.);
#8898=ORIENTED_EDGE('',*,*,#6676,.T.);
#8899=ORIENTED_EDGE('',*,*,#6591,.T.);
#8900=ORIENTED_EDGE('',*,*,#6657,.F.);
#8901=ORIENTED_EDGE('',*,*,#6637,.T.);
#8902=ORIENTED_EDGE('',*,*,#6622,.F.);
#8903=ORIENTED_EDGE('',*,*,#6564,.F.);
#8904=ORIENTED_EDGE('',*,*,#6685,.T.);
#8905=ORIENTED_EDGE('',*,*,#6677,.F.);
#8906=ORIENTED_EDGE('',*,*,#6667,.T.);
#8907=ORIENTED_EDGE('',*,*,#6686,.F.);
#8908=ORIENTED_EDGE('',*,*,#6687,.T.);
#8909=ORIENTED_EDGE('',*,*,#6688,.T.);
#8910=ORIENTED_EDGE('',*,*,#6672,.T.);
#8911=ORIENTED_EDGE('',*,*,#6684,.F.);
#8912=ORIENTED_EDGE('',*,*,#6679,.F.);
#8913=ORIENTED_EDGE('',*,*,#6647,.F.);
#8914=ORIENTED_EDGE('',*,*,#6626,.F.);
#8915=ORIENTED_EDGE('',*,*,#6607,.T.);
#8916=ORIENTED_EDGE('',*,*,#6605,.F.);
#8917=ORIENTED_EDGE('',*,*,#6580,.T.);
#8918=ORIENTED_EDGE('',*,*,#6651,.T.);
#8919=ORIENTED_EDGE('',*,*,#6653,.T.);
#8920=ORIENTED_EDGE('',*,*,#6649,.T.);
#8921=ORIENTED_EDGE('',*,*,#6631,.T.);
#8922=ORIENTED_EDGE('',*,*,#6644,.F.);
#8923=ORIENTED_EDGE('',*,*,#6635,.T.);
#8924=ORIENTED_EDGE('',*,*,#6655,.T.);
#8925=ORIENTED_EDGE('',*,*,#6563,.F.);
#8926=ORIENTED_EDGE('',*,*,#6577,.F.);
#8927=ORIENTED_EDGE('',*,*,#6678,.F.);
#8928=ORIENTED_EDGE('',*,*,#6685,.F.);
#8929=ORIENTED_EDGE('',*,*,#6583,.F.);
#8930=ORIENTED_EDGE('',*,*,#6599,.F.);
#8931=ORIENTED_EDGE('',*,*,#6681,.F.);
#8932=ORIENTED_EDGE('',*,*,#6616,.F.);
#8933=ORIENTED_EDGE('',*,*,#6688,.F.);
#8934=ORIENTED_EDGE('',*,*,#6689,.T.);
#8935=ORIENTED_EDGE('',*,*,#6658,.T.);
#8936=ORIENTED_EDGE('',*,*,#6690,.T.);
#8937=ORIENTED_EDGE('',*,*,#6594,.T.);
#8938=ORIENTED_EDGE('',*,*,#6673,.F.);
#8939=ORIENTED_EDGE('',*,*,#6596,.F.);
#8940=ORIENTED_EDGE('',*,*,#6691,.T.);
#8941=ORIENTED_EDGE('',*,*,#6660,.T.);
#8942=ORIENTED_EDGE('',*,*,#6692,.T.);
#8943=ORIENTED_EDGE('',*,*,#6686,.T.);
#8944=ORIENTED_EDGE('',*,*,#6666,.F.);
#8945=ORIENTED_EDGE('',*,*,#6662,.F.);
#8946=ORIENTED_EDGE('',*,*,#6574,.F.);
#8947=ORIENTED_EDGE('',*,*,#6670,.F.);
#8948=ORIENTED_EDGE('',*,*,#6682,.F.);
#8949=ORIENTED_EDGE('',*,*,#6664,.F.);
#8950=ORIENTED_EDGE('',*,*,#6683,.F.);
#8951=ORIENTED_EDGE('',*,*,#6675,.F.);
#8952=ORIENTED_EDGE('',*,*,#6619,.F.);
#8953=ORIENTED_EDGE('',*,*,#6692,.F.);
#8954=ORIENTED_EDGE('',*,*,#6659,.F.);
#8955=ORIENTED_EDGE('',*,*,#6689,.F.);
#8956=ORIENTED_EDGE('',*,*,#6687,.F.);
#8957=ORIENTED_EDGE('',*,*,#6691,.F.);
#8958=ORIENTED_EDGE('',*,*,#6595,.F.);
#8959=ORIENTED_EDGE('',*,*,#6690,.F.);
#8960=ORIENTED_EDGE('',*,*,#6661,.F.);
#11283=CONICAL_SURFACE('',#12694,14.7,0.785398163397379);
#11284=CONICAL_SURFACE('',#12697,15.,0.785398163397457);
#11492=ADVANCED_FACE('',(#1410),#1048,.T.);
#11493=ADVANCED_FACE('',(#1411,#363,#364),#514,.F.);
#11494=ADVANCED_FACE('',(#1412),#515,.F.);
#11495=ADVANCED_FACE('',(#1413),#1049,.T.);
#11496=ADVANCED_FACE('',(#1414,#365,#366,#367),#516,.F.);
#11497=ADVANCED_FACE('',(#1415),#517,.F.);
#11498=ADVANCED_FACE('',(#1416),#1050,.F.);
#11499=ADVANCED_FACE('',(#1417),#518,.F.);
#11500=ADVANCED_FACE('',(#1418),#1051,.F.);
#11501=ADVANCED_FACE('',(#1419),#519,.F.);
#11502=ADVANCED_FACE('',(#1420),#520,.F.);
#11503=ADVANCED_FACE('',(#1421,#368,#369),#521,.T.);
#11504=ADVANCED_FACE('',(#1422),#522,.F.);
#11505=ADVANCED_FACE('',(#1423),#11283,.T.);
#11506=ADVANCED_FACE('',(#1424),#11284,.T.);
#11507=ADVANCED_FACE('',(#1425),#825,.F.);
#11508=ADVANCED_FACE('',(#1426),#826,.F.);
#11509=ADVANCED_FACE('',(#1427),#1052,.F.);
#11510=ADVANCED_FACE('',(#1428),#1053,.F.);
#11511=ADVANCED_FACE('',(#1429),#1054,.F.);
#11512=ADVANCED_FACE('',(#1430),#1055,.T.);
#11513=ADVANCED_FACE('',(#1431),#1056,.F.);
#11514=ADVANCED_FACE('',(#1432),#1057,.F.);
#11515=ADVANCED_FACE('',(#1433),#1058,.F.);
#11516=ADVANCED_FACE('',(#1434),#1059,.T.);
#11517=ADVANCED_FACE('',(#1435),#523,.F.);
#11518=ADVANCED_FACE('',(#1436),#1060,.T.);
#11519=ADVANCED_FACE('',(#1437),#1061,.T.);
#11520=ADVANCED_FACE('',(#1438),#524,.F.);
#11521=ADVANCED_FACE('',(#1439),#525,.F.);
#11522=ADVANCED_FACE('',(#1440),#526,.F.);
#11523=ADVANCED_FACE('',(#1441),#527,.F.);
#11524=ADVANCED_FACE('',(#1442),#528,.F.);
#11525=ADVANCED_FACE('',(#1443),#529,.F.);
#11526=ADVANCED_FACE('',(#1444),#530,.F.);
#11527=ADVANCED_FACE('',(#1445,#370,#371,#372),#531,.F.);
#11528=ADVANCED_FACE('',(#1446,#373),#532,.T.);
#11529=ADVANCED_FACE('',(#1447,#374),#533,.T.);
#11530=ADVANCED_FACE('',(#1448),#1062,.T.);
#11531=ADVANCED_FACE('',(#1449),#1063,.T.);
#11532=ADVANCED_FACE('',(#1450),#534,.T.);
#11533=ADVANCED_FACE('',(#1451),#535,.T.);
#11534=ADVANCED_FACE('',(#1452),#1064,.T.);
#11535=ADVANCED_FACE('',(#1453),#1065,.T.);
#11536=ADVANCED_FACE('',(#1454),#1066,.F.);
#11537=ADVANCED_FACE('',(#1455),#1067,.F.);
#12027=CLOSED_SHELL('',(#11492,#11493,#11494,#11495,#11496,#11497,#11498,
#11499,#11500,#11501,#11502,#11503,#11504,#11505,#11506,#11507,#11508,#11509,
#11510,#11511,#11512,#11513,#11514,#11515,#11516,#11517,#11518,#11519,#11520,
#11521,#11522,#11523,#11524,#11525,#11526,#11527,#11528,#11529,#11530,#11531,
#11532,#11533,#11534,#11535,#11536,#11537));
#12653=AXIS2_PLACEMENT_3D('',#18471,#14659,#14660);
#12654=AXIS2_PLACEMENT_3D('',#18472,#14661,#14662);
#12655=AXIS2_PLACEMENT_3D('',#18475,#14663,#14664);
#12656=AXIS2_PLACEMENT_3D('',#18479,#14666,#14667);
#12657=AXIS2_PLACEMENT_3D('',#18481,#14669,#14670);
#12658=AXIS2_PLACEMENT_3D('',#18485,#14672,#14673);
#12659=AXIS2_PLACEMENT_3D('',#18491,#14676,#14677);
#12660=AXIS2_PLACEMENT_3D('',#18497,#14680,#14681);
#12661=AXIS2_PLACEMENT_3D('',#18501,#14683,#14684);
#12662=AXIS2_PLACEMENT_3D('',#18504,#14686,#14687);
#12663=AXIS2_PLACEMENT_3D('',#18506,#14688,#14689);
#12664=AXIS2_PLACEMENT_3D('',#18508,#14690,#14691);
#12665=AXIS2_PLACEMENT_3D('',#18509,#14692,#14693);
#12666=AXIS2_PLACEMENT_3D('',#18513,#14696,#14697);
#12667=AXIS2_PLACEMENT_3D('',#18516,#14698,#14699);
#12668=AXIS2_PLACEMENT_3D('',#18520,#14701,#14702);
#12669=AXIS2_PLACEMENT_3D('',#18522,#14704,#14705);
#12670=AXIS2_PLACEMENT_3D('',#18526,#14707,#14708);
#12671=AXIS2_PLACEMENT_3D('',#18532,#14711,#14712);
#12672=AXIS2_PLACEMENT_3D('',#18538,#14715,#14716);
#12673=AXIS2_PLACEMENT_3D('',#18546,#14720,#14721);
#12674=AXIS2_PLACEMENT_3D('',#18549,#14723,#14724);
#12675=AXIS2_PLACEMENT_3D('',#18551,#14725,#14726);
#12676=AXIS2_PLACEMENT_3D('',#18553,#14727,#14728);
#12677=AXIS2_PLACEMENT_3D('',#18555,#14729,#14730);
#12678=AXIS2_PLACEMENT_3D('',#18556,#14731,#14732);
#12679=AXIS2_PLACEMENT_3D('',#18560,#14735,#14736);
#12680=AXIS2_PLACEMENT_3D('',#18562,#14737,#14738);
#12681=AXIS2_PLACEMENT_3D('',#18564,#14740,#14741);
#12682=AXIS2_PLACEMENT_3D('',#18568,#14744,#14745);
#12683=AXIS2_PLACEMENT_3D('',#18570,#14746,#14747);
#12684=AXIS2_PLACEMENT_3D('',#18572,#14749,#14750);
#12685=AXIS2_PLACEMENT_3D('',#18576,#14753,#14754);
#12686=AXIS2_PLACEMENT_3D('',#18589,#14757,#14758);
#12687=AXIS2_PLACEMENT_3D('',#18591,#14759,#14760);
#12688=AXIS2_PLACEMENT_3D('',#18595,#14762,#14763);
#12689=AXIS2_PLACEMENT_3D('',#18599,#14765,#14766);
#12690=AXIS2_PLACEMENT_3D('',#18604,#14769,#14770);
#12691=AXIS2_PLACEMENT_3D('',#18606,#14771,#14772);
#12692=AXIS2_PLACEMENT_3D('',#18608,#14773,#14774);
#12693=AXIS2_PLACEMENT_3D('',#18609,#14775,#14776);
#12694=AXIS2_PLACEMENT_3D('',#18618,#14779,#14780);
#12695=AXIS2_PLACEMENT_3D('',#18620,#14781,#14782);
#12696=AXIS2_PLACEMENT_3D('',#18623,#14784,#14785);
#12697=AXIS2_PLACEMENT_3D('',#18624,#14786,#14787);
#12698=AXIS2_PLACEMENT_3D('',#18627,#14788,#14789);
#12699=AXIS2_PLACEMENT_3D('',#18628,#14790,#14791);
#12700=AXIS2_PLACEMENT_3D('',#18631,#14793,#14794);
#12701=AXIS2_PLACEMENT_3D('',#18632,#14795,#14796);
#12702=AXIS2_PLACEMENT_3D('',#18634,#14797,#14798);
#12703=AXIS2_PLACEMENT_3D('',#18640,#14799,#14800);
#12704=AXIS2_PLACEMENT_3D('',#18641,#14801,#14802);
#12705=AXIS2_PLACEMENT_3D('',#18643,#14803,#14804);
#12706=AXIS2_PLACEMENT_3D('',#18645,#14805,#14806);
#12707=AXIS2_PLACEMENT_3D('',#18654,#14807,#14808);
#12708=AXIS2_PLACEMENT_3D('',#18656,#14810,#14811);
#12709=AXIS2_PLACEMENT_3D('',#18658,#14813,#14814);
#12710=AXIS2_PLACEMENT_3D('',#18660,#14815,#14816);
#12711=AXIS2_PLACEMENT_3D('',#18662,#14818,#14819);
#12712=AXIS2_PLACEMENT_3D('',#18665,#14821,#14822);
#12713=AXIS2_PLACEMENT_3D('',#18667,#14824,#14825);
#12714=AXIS2_PLACEMENT_3D('',#18669,#14826,#14827);
#12715=AXIS2_PLACEMENT_3D('',#18671,#14829,#14830);
#12716=AXIS2_PLACEMENT_3D('',#18673,#14831,#14832);
#12717=AXIS2_PLACEMENT_3D('',#18675,#14834,#14835);
#12718=AXIS2_PLACEMENT_3D('',#18677,#14836,#14837);
#12719=AXIS2_PLACEMENT_3D('',#18680,#14839,#14840);
#12720=AXIS2_PLACEMENT_3D('',#18681,#14841,#14842);
#12721=AXIS2_PLACEMENT_3D('',#18684,#14845,#14846);
#12722=AXIS2_PLACEMENT_3D('',#18693,#14851,#14852);
#12723=AXIS2_PLACEMENT_3D('',#18719,#14856,#14857);
#12724=AXIS2_PLACEMENT_3D('',#18721,#14859,#14860);
#12725=AXIS2_PLACEMENT_3D('',#18738,#14863,#14864);
#12726=AXIS2_PLACEMENT_3D('',#18751,#14867,#14868);
#12727=AXIS2_PLACEMENT_3D('',#18753,#14870,#14871);
#12728=AXIS2_PLACEMENT_3D('',#18757,#14874,#14875);
#12729=AXIS2_PLACEMENT_3D('',#18761,#14878,#14879);
#12730=AXIS2_PLACEMENT_3D('',#18763,#14881,#14882);
#12731=AXIS2_PLACEMENT_3D('',#18766,#14885,#14886);
#12732=AXIS2_PLACEMENT_3D('',#18768,#14888,#14889);
#12733=AXIS2_PLACEMENT_3D('',#18769,#14890,#14891);
#12734=AXIS2_PLACEMENT_3D('',#18770,#14892,#14893);
#12735=AXIS2_PLACEMENT_3D('',#18776,#14897,#14898);
#12736=AXIS2_PLACEMENT_3D('',#18777,#14899,#14900);
#12737=AXIS2_PLACEMENT_3D('',#18778,#14901,#14902);
#12738=AXIS2_PLACEMENT_3D('',#18779,#14903,#14904);
#12739=AXIS2_PLACEMENT_3D('',#18780,#14905,#14906);
#12740=AXIS2_PLACEMENT_3D('',#18781,#14907,#14908);
#12741=AXIS2_PLACEMENT_3D('',#18782,#14909,#14910);
#12742=AXIS2_PLACEMENT_3D('',#18783,#14911,#14912);
#12743=AXIS2_PLACEMENT_3D('',#18784,#14913,#14914);
#12744=AXIS2_PLACEMENT_3D('',#18785,#14915,#14916);
#12745=AXIS2_PLACEMENT_3D('',#18786,#14917,#14918);
#12746=AXIS2_PLACEMENT_3D('',#18787,#14919,#14920);
#12747=AXIS2_PLACEMENT_3D('',#18788,#14921,#14922);
#12748=AXIS2_PLACEMENT_3D('',#18789,#14923,#14924);
#14659=DIRECTION('axis',(0.,0.,1.));
#14660=DIRECTION('refdir',(1.,0.,0.));
#14661=DIRECTION('center_axis',(0.,0.,1.));
#14662=DIRECTION('ref_axis',(0.723913745035715,0.689890491127661,0.));
#14663=DIRECTION('center_axis',(9.49460883474904E-17,-8.60566842858052E-17,
1.));
#14664=DIRECTION('ref_axis',(0.723913745035715,0.689890491127661,0.));
#14665=DIRECTION('',(0.,0.,1.));
#14666=DIRECTION('center_axis',(-9.47278923080924E-17,-4.21179355246917E-17,
-1.));
#14667=DIRECTION('ref_axis',(0.723913745035715,0.689890491127661,0.));
#14668=DIRECTION('',(0.,0.,-1.));
#14669=DIRECTION('center_axis',(9.49460883474904E-17,-8.60566842858052E-17,
1.));
#14670=DIRECTION('ref_axis',(0.999998551032278,0.00170233173745095,-9.47994537487936E-17));
#14671=DIRECTION('',(-0.689890491127661,0.723913745035715,1.27800020127394E-16));
#14672=DIRECTION('center_axis',(-9.49460883474904E-17,8.60566842858052E-17,
-1.));
#14673=DIRECTION('ref_axis',(0.444137634660357,0.89595857129574,0.));
#14674=DIRECTION('',(-0.993849755374348,0.110736912284699,1.03891798177174E-16));
#14675=DIRECTION('',(0.981518914375337,-0.191365150232375,-1.09659631875867E-16));
#14676=DIRECTION('center_axis',(9.49460883474904E-17,-8.60566842858052E-17,
1.));
#14677=DIRECTION('ref_axis',(0.999998551032278,0.00170233173745172,-9.47994537487935E-17));
#14678=DIRECTION('',(-0.984295785396816,-0.176527071153592,7.82637001701861E-17));
#14679=DIRECTION('',(0.00170233173745037,-0.999998551032278,-8.62181893319881E-17));
#14680=DIRECTION('center_axis',(-9.49460883474904E-17,8.60566842858052E-17,
-1.));
#14681=DIRECTION('ref_axis',(0.999998551032278,0.00170233173744927,-9.47994537487937E-17));
#14682=DIRECTION('',(0.999998551032278,0.00170233173745092,-9.47994537487935E-17));
#14683=DIRECTION('center_axis',(-9.49460883474904E-17,8.60566842858052E-17,
-1.));
#14684=DIRECTION('ref_axis',(0.999998551032278,0.00170233173744834,-9.47994537487938E-17));
#14685=DIRECTION('',(-0.175324395549563,0.984510719253569,1.01370093692115E-16));
#14686=DIRECTION('center_axis',(-9.49460883474904E-17,8.60566842858052E-17,
-1.));
#14687=DIRECTION('ref_axis',(0.999998551032278,0.00170233173745093,-9.47994537487936E-17));
#14688=DIRECTION('center_axis',(9.49460883474904E-17,-8.60566842858052E-17,
1.));
#14689=DIRECTION('ref_axis',(0.999998551032278,0.00170233173744927,-9.47994537487937E-17));
#14690=DIRECTION('center_axis',(9.49460883474904E-17,-8.60566842858052E-17,
1.));
#14691=DIRECTION('ref_axis',(0.999998551032278,0.00170233173745053,-9.47994537487936E-17));
#14692=DIRECTION('center_axis',(0.723913745035715,0.689890491127661,0.));
#14693=DIRECTION('ref_axis',(0.689890491127661,-0.723913745035715,0.));
#14694=DIRECTION('',(0.689890491127661,-0.723913745035715,-3.48621197090657E-17));
#14695=DIRECTION('',(0.,0.,1.));
#14696=DIRECTION('center_axis',(0.,0.,1.));
#14697=DIRECTION('ref_axis',(0.723913745035715,0.689890491127661,0.));
#14698=DIRECTION('center_axis',(9.47278923080924E-17,4.21179355246917E-17,
1.));
#14699=DIRECTION('ref_axis',(0.723913745035715,0.689890491127661,0.));
#14700=DIRECTION('',(0.,0.,1.));
#14701=DIRECTION('center_axis',(-9.49460883474904E-17,8.60566842858052E-17,
-1.));
#14702=DIRECTION('ref_axis',(0.723913745035715,0.689890491127661,0.));
#14703=DIRECTION('',(0.,0.,-1.));
#14704=DIRECTION('center_axis',(9.47278923080924E-17,4.21179355246917E-17,
1.));
#14705=DIRECTION('ref_axis',(0.00170233173745095,-0.999998551032278,4.19566161996647E-17));
#14706=DIRECTION('',(-0.689890491127661,0.723913745035715,3.48621197090657E-17));
#14707=DIRECTION('center_axis',(-9.47278923080924E-17,-4.21179355246917E-17,
-1.));
#14708=DIRECTION('ref_axis',(0.444137634660357,0.89595857129574,0.));
#14709=DIRECTION('',(-0.993849755374348,0.110736912284699,8.94812824657148E-17));
#14710=DIRECTION('',(0.981518914375337,-0.191365150232375,-8.49173129601425E-17));
#14711=DIRECTION('center_axis',(9.47278923080924E-17,4.21179355246917E-17,
1.));
#14712=DIRECTION('ref_axis',(0.00170233173745019,-0.999998551032278,4.19566161996648E-17));
#14713=DIRECTION('',(-0.984295785396816,-0.176527071153591,1.00675220959588E-16));
#14714=DIRECTION('',(0.00170233173745037,-0.999998551032278,4.19566161996648E-17));
#14715=DIRECTION('center_axis',(-9.47278923080924E-17,-4.21179355246917E-17,
-1.));
#14716=DIRECTION('ref_axis',(0.00170233173744927,-0.999998551032278,4.19566161996649E-17));
#14717=DIRECTION('',(-0.00170233173745037,0.999998551032278,8.62181893319882E-17));
#14718=DIRECTION('',(0.999998551032278,0.00170233173745037,-9.47994537487936E-17));
#14719=DIRECTION('',(-0.00170233173745037,0.999998551032278,8.62181893319881E-17));
#14720=DIRECTION('center_axis',(-9.47278923080924E-17,-4.21179355246917E-17,
-1.));
#14721=DIRECTION('ref_axis',(0.00170233173745089,-0.999998551032278,4.19566161996647E-17));
#14722=DIRECTION('',(-0.175324395549563,0.984510719253569,-2.48574485362892E-17));
#14723=DIRECTION('center_axis',(-9.47278923080924E-17,-4.21179355246917E-17,
-1.));
#14724=DIRECTION('ref_axis',(0.00170233173745093,-0.999998551032278,4.19566161996647E-17));
#14725=DIRECTION('center_axis',(9.47278923080924E-17,4.21179355246917E-17,
1.));
#14726=DIRECTION('ref_axis',(0.00170233173745116,-0.999998551032278,4.19566161996647E-17));
#14727=DIRECTION('center_axis',(9.47278923080924E-17,4.21179355246917E-17,
1.));
#14728=DIRECTION('ref_axis',(0.00170233173744927,-0.999998551032278,4.19566161996649E-17));
#14729=DIRECTION('center_axis',(9.47278923080924E-17,4.21179355246917E-17,
1.));
#14730=DIRECTION('ref_axis',(0.00170233173745101,-0.999998551032278,4.19566161996647E-17));
#14731=DIRECTION('center_axis',(0.723913745035715,0.689890491127661,0.));
#14732=DIRECTION('ref_axis',(0.689890491127661,-0.723913745035715,0.));
#14733=DIRECTION('',(0.689890491127661,-0.723913745035715,-1.27800020127394E-16));
#14734=DIRECTION('',(0.,0.,1.));
#14735=DIRECTION('center_axis',(0.,0.,-1.));
#14736=DIRECTION('ref_axis',(0.444137634660357,0.89595857129574,0.));
#14737=DIRECTION('center_axis',(9.47278923080924E-17,4.21179355246917E-17,
1.));
#14738=DIRECTION('ref_axis',(0.444137634660357,0.89595857129574,0.));
#14739=DIRECTION('',(0.,0.,-1.));
#14740=DIRECTION('center_axis',(0.110736912284699,0.993849755374348,0.));
#14741=DIRECTION('ref_axis',(0.993849755374348,-0.110736912284699,0.));
#14742=DIRECTION('',(0.993849755374348,-0.110736912284699,-8.94812824657148E-17));
#14743=DIRECTION('',(-8.08477301668617E-16,9.00823082713598E-17,1.));
#14744=DIRECTION('center_axis',(0.,0.,-1.));
#14745=DIRECTION('ref_axis',(0.444137634660357,0.89595857129574,0.));
#14746=DIRECTION('center_axis',(9.49460883474904E-17,-8.60566842858052E-17,
1.));
#14747=DIRECTION('ref_axis',(0.444137634660357,0.89595857129574,0.));
#14748=DIRECTION('',(0.,0.,-1.));
#14749=DIRECTION('center_axis',(0.110736912284699,0.993849755374348,0.));
#14750=DIRECTION('ref_axis',(0.993849755374348,-0.110736912284699,0.));
#14751=DIRECTION('',(0.993849755374348,-0.110736912284699,-1.03891798177174E-16));
#14752=DIRECTION('',(-8.08477301668617E-16,9.00823082713598E-17,1.));
#14753=DIRECTION('center_axis',(0.191365150232375,0.981518914375337,6.62968908743508E-17));
#14754=DIRECTION('ref_axis',(-0.981518914375337,0.191365150232375,1.09659631875867E-16));
#14755=DIRECTION('',(0.981518914375337,-0.191365150232375,-1.09659631875867E-16));
#14756=DIRECTION('',(-9.49460883474904E-17,8.60566842858052E-17,-1.));
#14757=DIRECTION('center_axis',(9.49460883474904E-17,-8.60566842858052E-17,
1.));
#14758=DIRECTION('ref_axis',(0.999998551032278,0.00170233173745095,-9.47994537487936E-17));
#14759=DIRECTION('center_axis',(9.49460883474904E-17,-8.60566842858052E-17,
1.));
#14760=DIRECTION('ref_axis',(0.999998551032278,0.00170233173745093,-9.47994537487936E-17));
#14761=DIRECTION('',(-0.175324395549563,0.984510719253569,1.01370093692115E-16));
#14762=DIRECTION('center_axis',(9.49460883474904E-17,-8.60566842858052E-17,
1.));
#14763=DIRECTION('ref_axis',(0.999998551032278,0.00170233173745112,-9.47994537487936E-17));
#14764=DIRECTION('',(-0.999998551032278,-0.00170233173745092,9.47994537487935E-17));
#14765=DIRECTION('center_axis',(9.49460883474904E-17,-8.60566842858052E-17,
1.));
#14766=DIRECTION('ref_axis',(0.999998551032278,0.00170233173744927,-9.47994537487937E-17));
#14767=DIRECTION('',(0.00170233173745037,-0.999998551032278,-8.62181893319881E-17));
#14768=DIRECTION('',(-0.984295785396816,-0.176527071153592,7.82637001701861E-17));
#14769=DIRECTION('center_axis',(-9.49460883474904E-17,8.60566842858052E-17,
-1.));
#14770=DIRECTION('ref_axis',(0.999998551032278,0.00170233173744519,-9.47994537487941E-17));
#14771=DIRECTION('center_axis',(9.49460883474904E-17,-8.60566842858052E-17,
1.));
#14772=DIRECTION('ref_axis',(0.999998551032278,0.00170233173745053,-9.47994537487936E-17));
#14773=DIRECTION('center_axis',(9.49460883474904E-17,-8.60566842858052E-17,
1.));
#14774=DIRECTION('ref_axis',(0.999998551032278,0.00170233173744927,-9.47994537487937E-17));
#14775=DIRECTION('center_axis',(0.191365150232375,0.981518914375337,6.62968908743508E-17));
#14776=DIRECTION('ref_axis',(-0.981518914375337,0.191365150232375,1.09659631875867E-16));
#14777=DIRECTION('',(-0.981518914375337,0.191365150232375,8.49173129601425E-17));
#14778=DIRECTION('',(-9.49460883474904E-17,8.60566842858052E-17,-1.));
#14779=DIRECTION('center_axis',(-9.49460883474904E-17,8.60566842858052E-17,
-1.));
#14780=DIRECTION('ref_axis',(-0.999998551032278,-0.00170233173745069,9.47994537487936E-17));
#14781=DIRECTION('center_axis',(-9.49460883474904E-17,8.60566842858052E-17,
-1.));
#14782=DIRECTION('ref_axis',(0.999998551032278,0.00170233173745204,-9.47994537487934E-17));
#14783=DIRECTION('',(-0.707105756611597,-0.00120373031538035,0.707106781186597));
#14784=DIRECTION('center_axis',(9.49460883474904E-17,-8.60566842858052E-17,
1.));
#14785=DIRECTION('ref_axis',(0.999998551032278,0.00170233173745069,-9.47994537487936E-17));
#14786=DIRECTION('center_axis',(9.49460883474904E-17,-8.60566842858052E-17,
1.));
#14787=DIRECTION('ref_axis',(0.999998551032278,0.00170233173745019,-9.47994537487936E-17));
#14788=DIRECTION('center_axis',(9.49460883474904E-17,-8.60566842858052E-17,
1.));
#14789=DIRECTION('ref_axis',(-0.999998551032278,-0.00170233173745204,9.47994537487934E-17));
#14790=DIRECTION('center_axis',(9.49460883474904E-17,-8.60566842858052E-17,
1.));
#14791=DIRECTION('ref_axis',(-0.999998551032278,-0.00170233173745204,9.47994537487934E-17));
#14792=DIRECTION('',(0.707105756611652,0.00120373031538027,-0.707106781186541));
#14793=DIRECTION('center_axis',(-9.49460883474904E-17,8.60566842858052E-17,
-1.));
#14794=DIRECTION('ref_axis',(-0.999998551032278,-0.00170233173745068,9.47994537487936E-17));
#14795=DIRECTION('center_axis',(9.49460883474904E-17,-8.60566842858052E-17,
1.));
#14796=DIRECTION('ref_axis',(0.999998551032278,0.00170233173745104,0.));
#14797=DIRECTION('center_axis',(9.49460883474904E-17,-8.60566842858052E-17,
1.));
#14798=DIRECTION('ref_axis',(0.999998551032278,0.00170233173745019,-9.47994537487936E-17));
#14799=DIRECTION('center_axis',(9.49460883474904E-17,-8.60566842858052E-17,
1.));
#14800=DIRECTION('ref_axis',(0.999998551032278,0.00170233173745019,-9.47994537487936E-17));
#14801=DIRECTION('center_axis',(9.49460883474904E-17,-8.60566842858052E-17,
1.));
#14802=DIRECTION('ref_axis',(0.999998551032278,0.00170233173745104,0.));
#14803=DIRECTION('center_axis',(-9.49460883474904E-17,8.60566842858052E-17,
-1.));
#14804=DIRECTION('ref_axis',(0.999998551032278,0.00170233173745019,-9.47994537487936E-17));
#14805=DIRECTION('center_axis',(-9.49460883474904E-17,8.60566842858052E-17,
-1.));
#14806=DIRECTION('ref_axis',(0.999998551032278,0.00170233173745019,-9.47994537487936E-17));
#14807=DIRECTION('center_axis',(-9.49460883474904E-17,8.60566842858052E-17,
-1.));
#14808=DIRECTION('ref_axis',(-0.999998551032278,-0.00170233173745053,9.47994537487936E-17));
#14809=DIRECTION('',(-9.49460883474904E-17,8.60566842858052E-17,-1.));
#14810=DIRECTION('center_axis',(-9.49460883474904E-17,8.60566842858052E-17,
-1.));
#14811=DIRECTION('ref_axis',(-0.999998551032278,-0.00170233173744927,9.47994537487937E-17));
#14812=DIRECTION('',(-9.49460883474904E-17,8.60566842858052E-17,-1.));
#14813=DIRECTION('center_axis',(-9.49460883474904E-17,8.60566842858052E-17,
-1.));
#14814=DIRECTION('ref_axis',(-0.999998551032278,-0.00170233173744927,9.47994537487937E-17));
#14815=DIRECTION('center_axis',(9.49460883474904E-17,-8.60566842858052E-17,
1.));
#14816=DIRECTION('ref_axis',(0.999998551032278,0.00170233173744927,-9.47994537487937E-17));
#14817=DIRECTION('',(-9.49460883474904E-17,8.60566842858052E-17,-1.));
#14818=DIRECTION('center_axis',(-9.49460883474904E-17,8.60566842858052E-17,
-1.));
#14819=DIRECTION('ref_axis',(-0.999998551032278,-0.00170233173745019,9.47994537487936E-17));
#14820=DIRECTION('',(9.49460883474904E-17,-8.60566842858052E-17,1.));
#14821=DIRECTION('center_axis',(-9.47278923080924E-17,-4.21179355246917E-17,
-1.));
#14822=DIRECTION('ref_axis',(-0.00170233173745019,0.999998551032278,-4.19566161996648E-17));
#14823=DIRECTION('',(-9.49460883474904E-17,8.60566842858052E-17,-1.));
#14824=DIRECTION('center_axis',(-9.49460883474904E-17,8.60566842858052E-17,
-1.));
#14825=DIRECTION('ref_axis',(-0.999998551032278,-0.00170233173745053,9.47994537487936E-17));
#14826=DIRECTION('center_axis',(-9.47278923080924E-17,-4.21179355246917E-17,
-1.));
#14827=DIRECTION('ref_axis',(-0.00170233173745115,0.999998551032278,-4.19566161996647E-17));
#14828=DIRECTION('',(-9.49460883474904E-17,8.60566842858052E-17,-1.));
#14829=DIRECTION('center_axis',(-9.49460883474904E-17,8.60566842858052E-17,
-1.));
#14830=DIRECTION('ref_axis',(-0.999998551032278,-0.00170233173744927,9.47994537487937E-17));
#14831=DIRECTION('center_axis',(-9.47278923080924E-17,-4.21179355246917E-17,
-1.));
#14832=DIRECTION('ref_axis',(-0.00170233173745101,0.999998551032278,-4.19566161996647E-17));
#14833=DIRECTION('',(-9.49460883474904E-17,8.60566842858052E-17,-1.));
#14834=DIRECTION('center_axis',(-9.49460883474904E-17,8.60566842858052E-17,
-1.));
#14835=DIRECTION('ref_axis',(-0.999998551032278,-0.00170233173744927,9.47994537487937E-17));
#14836=DIRECTION('center_axis',(-9.47278923080924E-17,-4.21179355246917E-17,
-1.));
#14837=DIRECTION('ref_axis',(-0.00170233173744927,0.999998551032278,-4.19566161996649E-17));
#14838=DIRECTION('',(-9.49460883474904E-17,8.60566842858052E-17,-1.));
#14839=DIRECTION('center_axis',(9.49460883474904E-17,-8.60566842858052E-17,
1.));
#14840=DIRECTION('ref_axis',(0.999998551032278,0.00170233173744927,-9.47994537487937E-17));
#14841=DIRECTION('center_axis',(-9.49460883474904E-17,8.60566842858052E-17,
-1.));
#14842=DIRECTION('ref_axis',(-0.999998551032278,-0.00170233173745019,9.47994537487936E-17));
#14843=DIRECTION('',(9.49460883474904E-17,-8.60566842858052E-17,1.));
#14844=DIRECTION('',(-9.49460883474904E-17,8.60566842858052E-17,-1.));
#14845=DIRECTION('center_axis',(-0.00170233173745037,0.999998551032278,
8.62181893319881E-17));
#14846=DIRECTION('ref_axis',(-0.999998551032278,-0.00170233173745037,9.47994537487936E-17));
#14847=DIRECTION('',(3.42763368692988E-16,-8.56348164531116E-17,1.));
#14848=DIRECTION('',(0.999998551032278,0.00170233173745037,-9.47994537487936E-17));
#14849=DIRECTION('',(-9.49460883474904E-17,8.60566842858052E-17,-1.));
#14850=DIRECTION('',(-0.999998551032278,-0.00170233173745037,9.47994537487936E-17));
#14851=DIRECTION('center_axis',(-9.49460883474904E-17,8.60566842858052E-17,
-1.));
#14852=DIRECTION('ref_axis',(-0.999998551032278,-0.00170233173745112,9.47994537487936E-17));
#14853=DIRECTION('',(-9.49460883474904E-17,8.60566842858052E-17,-1.));
#14854=DIRECTION('',(9.49460883474904E-17,-8.60566842858052E-17,1.));
#14855=DIRECTION('',(-9.49460883474904E-17,8.60566842858052E-17,-1.));
#14856=DIRECTION('center_axis',(9.47278923080924E-17,4.21179355246917E-17,
1.));
#14857=DIRECTION('ref_axis',(-0.00170233173744927,0.999998551032278,-4.19566161996649E-17));
#14858=DIRECTION('',(9.49460883474904E-17,-8.60566842858052E-17,1.));
#14859=DIRECTION('center_axis',(-9.49460883474904E-17,8.60566842858052E-17,
-1.));
#14860=DIRECTION('ref_axis',(-0.999998551032278,-0.00170233173744927,9.47994537487937E-17));
#14861=DIRECTION('',(9.49460883474904E-17,-8.60566842858052E-17,1.));
#14862=DIRECTION('',(-9.49460883474904E-17,8.60566842858052E-17,-1.));
#14863=DIRECTION('center_axis',(9.47278923080924E-17,4.21179355246917E-17,
1.));
#14864=DIRECTION('ref_axis',(-0.00170233173745274,0.999998551032278,-4.19566161996646E-17));
#14865=DIRECTION('',(9.49460883474904E-17,-8.60566842858052E-17,1.));
#14866=DIRECTION('',(-9.49460883474904E-17,8.60566842858052E-17,-1.));
#14867=DIRECTION('center_axis',(0.999998551032278,0.00170233173745037,-9.47994537487936E-17));
#14868=DIRECTION('ref_axis',(-0.00170233173745037,0.999998551032278,8.62181893319882E-17));
#14869=DIRECTION('',(-9.49460883474904E-17,8.60566842858052E-17,-1.));
#14870=DIRECTION('center_axis',(-0.984510719253569,-0.175324395549563,7.83876055738923E-17));
#14871=DIRECTION('ref_axis',(0.175324395549563,-0.984510719253569,-1.01370093692115E-16));
#14872=DIRECTION('',(0.175324395549563,-0.984510719253569,2.48574485362892E-17));
#14873=DIRECTION('',(-9.49460883474904E-17,8.60566842858052E-17,-1.));
#14874=DIRECTION('center_axis',(0.176527071153592,-0.984295785396816,-1.01465786541215E-16));
#14875=DIRECTION('ref_axis',(0.984295785396816,0.176527071153592,-7.8263700170186E-17));
#14876=DIRECTION('',(0.984295785396816,0.176527071153591,-1.00675220959588E-16));
#14877=DIRECTION('',(-9.49460883474904E-17,8.60566842858052E-17,-1.));
#14878=DIRECTION('center_axis',(-0.984510719253569,-0.175324395549563,7.83876055738923E-17));
#14879=DIRECTION('ref_axis',(0.175324395549563,-0.984510719253569,-1.01370093692115E-16));
#14880=DIRECTION('',(-9.49460883474904E-17,8.60566842858052E-17,-1.));
#14881=DIRECTION('center_axis',(0.00170233173745092,-0.999998551032278,
-8.62181893319882E-17));
#14882=DIRECTION('ref_axis',(0.999998551032278,0.00170233173745092,-9.47994537487936E-17));
#14883=DIRECTION('',(-0.999998551032278,-0.00170233173745092,9.47994537487935E-17));
#14884=DIRECTION('',(0.999998551032278,0.00170233173745092,-9.47994537487935E-17));
#14885=DIRECTION('center_axis',(0.999998551032278,0.00170233173745037,-9.47994537487936E-17));
#14886=DIRECTION('ref_axis',(-0.00170233173745037,0.999998551032278,8.62181893319882E-17));
#14887=DIRECTION('',(-0.00170233173745037,0.999998551032278,-4.19566161996648E-17));
#14888=DIRECTION('center_axis',(0.176527071153592,-0.984295785396816,-1.01465786541215E-16));
#14889=DIRECTION('ref_axis',(0.984295785396816,0.176527071153592,-7.8263700170186E-17));
#14890=DIRECTION('center_axis',(-9.47278923080924E-17,-4.21179355246917E-17,
-1.));
#14891=DIRECTION('ref_axis',(-0.00170233173745095,0.999998551032278,-4.19566161996647E-17));
#14892=DIRECTION('center_axis',(9.47278923080924E-17,4.21179355246917E-17,
1.));
#14893=DIRECTION('ref_axis',(-0.00170233173745177,0.999998551032278,-4.19566161996647E-17));
#14894=DIRECTION('',(-0.00170233173745037,0.999998551032278,8.62181893319881E-17));
#14895=DIRECTION('',(-0.999998551032278,-0.00170233173745037,9.47994537487936E-17));
#14896=DIRECTION('',(-0.00170233173745037,0.999998551032278,8.62181893319882E-17));
#14897=DIRECTION('center_axis',(9.49460883474904E-17,-8.60566842858052E-17,
1.));
#14898=DIRECTION('ref_axis',(0.999998551032278,0.00170233173745095,-9.47994537487936E-17));
#14899=DIRECTION('center_axis',(-9.49460883474904E-17,8.60566842858052E-17,
-1.));
#14900=DIRECTION('ref_axis',(0.999998551032278,0.00170233173745095,-9.47994537487936E-17));
#14901=DIRECTION('center_axis',(-9.49460883474904E-17,8.60566842858052E-17,
-1.));
#14902=DIRECTION('ref_axis',(0.807462267669275,-0.589919220139836,-1.27431875885094E-16));
#14903=DIRECTION('center_axis',(-9.49460883474904E-17,8.60566842858052E-17,
-1.));
#14904=DIRECTION('ref_axis',(0.807462267669275,-0.589919220139835,-1.27431875885094E-16));
#14905=DIRECTION('center_axis',(-0.999998551032278,-0.00170233173745037,
3.42617093174052E-16));
#14906=DIRECTION('ref_axis',(0.00170233173745037,-0.999998551032278,-8.62181893319881E-17));
#14907=DIRECTION('center_axis',(0.999998551032278,0.00170233173745037,-3.42617093174052E-16));
#14908=DIRECTION('ref_axis',(0.00170233173745037,-0.999998551032278,-3.76615600624924E-31));
#14909=DIRECTION('center_axis',(0.999998551032278,0.00170233173745037,-3.42617093174052E-16));
#14910=DIRECTION('ref_axis',(0.00170233173745037,-0.999998551032278,-3.76615600624924E-31));
#14911=DIRECTION('center_axis',(0.999998551032278,0.00170233173745037,-9.47994537487936E-17));
#14912=DIRECTION('ref_axis',(-0.00170233173745037,0.999998551032278,8.62181893319882E-17));
#14913=DIRECTION('center_axis',(-0.999998551032278,-0.00170233173745037,
9.47994537487936E-17));
#14914=DIRECTION('ref_axis',(-0.00170233173745037,0.999998551032278,1.04216884115654E-31));
#14915=DIRECTION('center_axis',(-0.999998551032278,-0.00170233173745037,
9.47994537487936E-17));
#14916=DIRECTION('ref_axis',(-0.00170233173745037,0.999998551032278,1.04216884115654E-31));
#14917=DIRECTION('center_axis',(-0.999998551032278,-0.00170233173745092,
9.47994537487936E-17));
#14918=DIRECTION('ref_axis',(0.00170233173745092,-0.999998551032278,1.06889111913492E-31));
#14919=DIRECTION('center_axis',(0.999998551032278,0.00170233173745092,-9.47994537487936E-17));
#14920=DIRECTION('ref_axis',(-0.00170233173745092,0.999998551032278,-1.06889111913492E-31));
#14921=DIRECTION('center_axis',(0.999998551032278,0.00170233173745037,-9.47994537487936E-17));
#14922=DIRECTION('ref_axis',(-0.00170233173745037,0.999998551032278,1.04216884115654E-31));
#14923=DIRECTION('center_axis',(0.999998551032278,0.00170233173745037,-9.47994537487936E-17));
#14924=DIRECTION('ref_axis',(-0.00170233173745037,0.999998551032278,1.04216884115654E-31));
#18471=CARTESIAN_POINT('',(0.,0.,0.));
#18472=CARTESIAN_POINT('Origin',(46.4876128454249,129.573387746387,272.073593133701));
#18473=CARTESIAN_POINT('',(30.1995535821213,114.050851696014,234.073593133701));
#18474=CARTESIAN_POINT('',(49.4633471679037,107.271033493035,234.073593133701));
#18475=CARTESIAN_POINT('Origin',(46.4876128454249,129.573387746387,234.073593133701));
#18476=CARTESIAN_POINT('',(49.4633471679037,107.271033493035,239.073593133701));
#18477=CARTESIAN_POINT('',(49.4633471679037,107.271033493035,272.073593133701));
#18478=CARTESIAN_POINT('',(30.1995535821213,114.050851696014,239.073593133701));
#18479=CARTESIAN_POINT('Origin',(46.4876128454249,129.573387746387,239.073593133701));
#18480=CARTESIAN_POINT('',(30.1995535821213,114.050851696014,272.073593133701));
#18481=CARTESIAN_POINT('Origin',(-232.939627118345,176.278148255689,234.073593133701));
#18482=CARTESIAN_POINT('',(28.8182642450608,115.50026192826,234.073593133701));
#18483=CARTESIAN_POINT('',(-55.5594395041075,204.039211666113,234.073593133701));
#18484=CARTESIAN_POINT('',(-4.90646155624503,132.218021461828,234.073593133701));
#18485=CARTESIAN_POINT('Origin',(-10.9969917319035,77.5562849162387,234.073593133701));
#18486=CARTESIAN_POINT('',(-192.605807708699,153.131892918133,234.073593133701));
#18487=CARTESIAN_POINT('',(-213.799107820696,155.493296744853,234.073593133701));
#18488=CARTESIAN_POINT('',(-227.957953056828,160.0244433382,234.073593133701));
#18489=CARTESIAN_POINT('',(77.1627332513468,100.535558183572,234.073593133701));
#18490=CARTESIAN_POINT('',(-227.713166902474,192.45480160587,234.073593133701));
#18491=CARTESIAN_POINT('Origin',(-232.939627118345,176.278148255689,234.073593133701));
#18492=CARTESIAN_POINT('',(-177.982268468343,201.373715997924,234.073593133701));
#18493=CARTESIAN_POINT('',(-235.587533185649,191.042585036641,234.073593133701));
#18494=CARTESIAN_POINT('',(-177.989077795293,205.373710202053,234.073593133701));
#18495=CARTESIAN_POINT('',(-177.982268468343,201.373715997924,234.073593133701));
#18496=CARTESIAN_POINT('',(-177.41038412351,208.374699678994,234.073593133701));
#18497=CARTESIAN_POINT('Origin',(-169.989089387034,205.387328855953,234.073593133701));
#18498=CARTESIAN_POINT('',(48.4156221649759,208.759131013669,234.073593133701));
#18499=CARTESIAN_POINT('',(-232.99410509728,208.28007760959,234.073593133701));
#18500=CARTESIAN_POINT('',(61.4104021126536,188.99066912614,234.073593133701));
#18501=CARTESIAN_POINT('Origin',(31.8750805350466,183.730937259653,234.073593133701));
#18502=CARTESIAN_POINT('',(70.7697436798221,136.43453699661,234.073593133701));
#18503=CARTESIAN_POINT('',(56.9969630433931,213.773746568613,234.073593133701));
#18504=CARTESIAN_POINT('Origin',(46.1569756984829,132.05142710787,234.073593133701));
#18505=CARTESIAN_POINT('',(45.0412410561795,187.753356260924,234.073593133701));
#18506=CARTESIAN_POINT('Origin',(37.0412526479213,187.739737607024,234.073593133701));
#18507=CARTESIAN_POINT('',(54.6251789940657,132.579591357641,234.073593133701));
#18508=CARTESIAN_POINT('Origin',(43.6251949327106,132.560865708529,234.073593133701));
#18509=CARTESIAN_POINT('Origin',(15.,130.,272.073593133701));
#18510=CARTESIAN_POINT('',(28.8182642450609,115.50026192826,239.073593133701));
#18511=CARTESIAN_POINT('',(10.0701475636351,135.172977429866,239.073593133701));
#18512=CARTESIAN_POINT('',(28.8182642450609,115.50026192826,272.073593133701));
#18513=CARTESIAN_POINT('Origin',(46.4876128454249,129.573387746387,272.073593133701));
#18514=CARTESIAN_POINT('',(30.1995535821213,114.050851696014,267.073593133701));
#18515=CARTESIAN_POINT('',(49.4633471679037,107.271033493035,267.073593133701));
#18516=CARTESIAN_POINT('Origin',(46.4876128454249,129.573387746387,267.073593133701));
#18517=CARTESIAN_POINT('',(49.4633471679037,107.271033493035,272.073593133701));
#18518=CARTESIAN_POINT('',(49.4633471679037,107.271033493035,272.073593133701));
#18519=CARTESIAN_POINT('',(30.1995535821213,114.050851696014,272.073593133701));
#18520=CARTESIAN_POINT('Origin',(46.4876128454249,129.573387746387,272.073593133701));
#18521=CARTESIAN_POINT('',(30.1995535821213,114.050851696014,272.073593133701));
#18522=CARTESIAN_POINT('Origin',(76.9784177883129,208.807754437623,267.073593133701));
#18523=CARTESIAN_POINT('',(28.8182642450609,115.50026192826,267.073593133701));
#18524=CARTESIAN_POINT('',(10.0701475636351,135.172977429866,267.073593133701));
#18525=CARTESIAN_POINT('',(-4.90646155624504,132.218021461828,267.073593133701));
#18526=CARTESIAN_POINT('Origin',(-10.9969917319035,77.5562849162387,267.073593133701));
#18527=CARTESIAN_POINT('',(-192.605807708699,153.131892918133,267.073593133701));
#18528=CARTESIAN_POINT('',(-62.5303325346189,138.638599131169,267.073593133701));
#18529=CARTESIAN_POINT('',(-235.81010437183,161.555364540059,267.073593133701));
#18530=CARTESIAN_POINT('',(77.1627332513468,100.535558183572,267.073593133701));
#18531=CARTESIAN_POINT('',(-235.587533185649,191.042585036641,267.073593133701));
#18532=CARTESIAN_POINT('Origin',(-232.939627118345,176.278148255689,267.073593133701));
#18533=CARTESIAN_POINT('',(-177.982268468343,201.373715997924,267.073593133701));
#18534=CARTESIAN_POINT('',(-235.587533185649,191.042585036641,267.073593133701));
#18535=CARTESIAN_POINT('',(-177.989077795293,205.373710202053,267.073593133701));
#18536=CARTESIAN_POINT('',(-177.982268468343,201.373715997924,267.073593133701));
#18537=CARTESIAN_POINT('',(-175.415302813384,211.265781701023,267.073593133701));
#18538=CARTESIAN_POINT('Origin',(-169.989089387034,205.387328855953,267.073593133701));
#18539=CARTESIAN_POINT('',(-175.406982357971,206.378107240404,267.073593133701));
#18540=CARTESIAN_POINT('',(-175.23725350376,106.674503914668,267.073593133701));
#18541=CARTESIAN_POINT('',(46.4190297263865,206.75572924813,267.073593133701));
#18542=CARTESIAN_POINT('',(46.4190297263865,206.75572924813,267.073593133701));
#18543=CARTESIAN_POINT('',(46.4135532795135,209.972751416803,267.073593133701));
#18544=CARTESIAN_POINT('',(46.5887585805977,107.052125922394,267.073593133701));
#18545=CARTESIAN_POINT('',(61.4104021126536,188.99066912614,267.073593133701));
#18546=CARTESIAN_POINT('Origin',(31.8750805350466,183.730937259653,267.073593133701));
#18547=CARTESIAN_POINT('',(70.7697436798221,136.43453699661,267.073593133701));
#18548=CARTESIAN_POINT('',(56.9969630433931,213.773746568613,267.073593133701));
#18549=CARTESIAN_POINT('Origin',(46.1569756984829,132.05142710787,267.073593133701));
#18550=CARTESIAN_POINT('',(54.6251789940657,132.579591357641,267.073593133701));
#18551=CARTESIAN_POINT('Origin',(43.6251949327106,132.560865708529,267.073593133701));
#18552=CARTESIAN_POINT('',(-224.939638710086,176.291766909589,267.073593133701));
#18553=CARTESIAN_POINT('Origin',(-232.939627118345,176.278148255689,267.073593133701));
#18554=CARTESIAN_POINT('',(45.0412410561795,187.753356260924,267.073593133701));
#18555=CARTESIAN_POINT('Origin',(37.0412526479213,187.739737607024,267.073593133701));
#18556=CARTESIAN_POINT('Origin',(15.,130.,272.073593133701));
#18557=CARTESIAN_POINT('',(28.8182642450608,115.50026192826,272.073593133701));
#18558=CARTESIAN_POINT('',(-55.5594395041075,204.039211666113,272.073593133701));
#18559=CARTESIAN_POINT('',(28.8182642450609,115.50026192826,272.073593133701));
#18560=CARTESIAN_POINT('Origin',(-10.9969917319035,77.5562849162387,272.073593133701));
#18561=CARTESIAN_POINT('',(-4.90646155624504,132.218021461828,239.073593133701));
#18562=CARTESIAN_POINT('Origin',(-10.9969917319035,77.5562849162387,239.073593133701));
#18563=CARTESIAN_POINT('',(-4.90646155624505,132.218021461828,272.073593133701));
#18564=CARTESIAN_POINT('Origin',(-192.605807708699,153.131892918133,272.073593133701));
#18565=CARTESIAN_POINT('',(-192.605807708699,153.131892918133,239.073593133701));
#18566=CARTESIAN_POINT('',(-62.5303325346189,138.638599131169,239.073593133701));
#18567=CARTESIAN_POINT('',(-192.605807708699,153.131892918133,272.073593133701));
#18568=CARTESIAN_POINT('Origin',(-10.9969917319035,77.5562849162387,272.073593133701));
#18569=CARTESIAN_POINT('',(-4.90646155624503,132.218021461828,272.073593133701));
#18570=CARTESIAN_POINT('Origin',(-10.9969917319035,77.5562849162387,272.073593133701));
#18571=CARTESIAN_POINT('',(-4.90646155624505,132.218021461828,272.073593133701));
#18572=CARTESIAN_POINT('Origin',(-192.605807708699,153.131892918133,272.073593133701));
#18573=CARTESIAN_POINT('',(-192.605807708699,153.131892918133,272.073593133701));
#18574=CARTESIAN_POINT('',(-213.799107820696,155.493296744853,272.073593133701));
#18575=CARTESIAN_POINT('',(-192.605807708699,153.131892918133,272.073593133701));
#18576=CARTESIAN_POINT('Origin',(77.1627332513468,100.535558183572,272.073593133701));
#18577=CARTESIAN_POINT('',(-227.957953056828,160.0244433382,272.073593133701));
#18578=CARTESIAN_POINT('',(77.1627332513468,100.535558183572,272.073593133701));
#18579=CARTESIAN_POINT('',(-235.81010437183,161.555364540059,274.073593133701));
#18580=CARTESIAN_POINT('Ctrl Pts',(-227.957953056828,160.0244433382,272.073593133701));
#18581=CARTESIAN_POINT('Ctrl Pts',(-228.546093465915,160.139112119509,272.073593133701));
#18582=CARTESIAN_POINT('Ctrl Pts',(-229.187572714652,160.264180287842,272.136134864339));
#18583=CARTESIAN_POINT('Ctrl Pts',(-230.458368646174,160.511945308759,272.351265898181));
#18584=CARTESIAN_POINT('Ctrl Pts',(-231.087933232071,160.63469049461,272.502332384129));
#18585=CARTESIAN_POINT('Ctrl Pts',(-232.977506438015,161.003097516761,273.025168777333));
#18586=CARTESIAN_POINT('Ctrl Pts',(-234.523328491993,161.304483934547,273.594881913422));
#18587=CARTESIAN_POINT('Ctrl Pts',(-235.81010437183,161.555364540059,274.073593133701));
#18588=CARTESIAN_POINT('',(-235.81010437183,161.555364540059,272.073593133701));
#18589=CARTESIAN_POINT('Origin',(-232.939627118345,176.278148255689,272.073593133701));
#18590=CARTESIAN_POINT('',(70.7697436798221,136.43453699661,272.073593133701));
#18591=CARTESIAN_POINT('Origin',(46.1569756984829,132.05142710787,272.073593133701));
#18592=CARTESIAN_POINT('',(61.4104021126536,188.99066912614,272.073593133701));
#18593=CARTESIAN_POINT('',(56.9969630433931,213.773746568613,272.073593133701));
#18594=CARTESIAN_POINT('',(48.4156221649759,208.759131013669,272.073593133701));
#18595=CARTESIAN_POINT('Origin',(31.8750805350466,183.730937259653,272.073593133701));
#18596=CARTESIAN_POINT('',(-177.41038412351,208.374699678994,272.073593133701));
#18597=CARTESIAN_POINT('',(-169.994196382247,208.38732450905,272.073593133701));
#18598=CARTESIAN_POINT('',(-177.989077795293,205.373710202053,272.073593133701));
#18599=CARTESIAN_POINT('Origin',(-169.989089387034,205.387328855953,272.073593133701));
#18600=CARTESIAN_POINT('',(-177.982268468343,201.373715997924,272.073593133701));
#18601=CARTESIAN_POINT('',(-177.982268468343,201.373715997924,272.073593133701));
#18602=CARTESIAN_POINT('',(-227.713166902474,192.45480160587,272.073593133701));
#18603=CARTESIAN_POINT('',(-235.587533185649,191.042585036641,272.073593133701));
#18604=CARTESIAN_POINT('Origin',(-232.939627118345,176.278148255689,272.073593133701));
#18605=CARTESIAN_POINT('',(54.6251789940657,132.579591357641,272.073593133701));
#18606=CARTESIAN_POINT('Origin',(43.6251949327106,132.560865708529,272.073593133701));
#18607=CARTESIAN_POINT('',(45.0412410561795,187.753356260924,272.073593133701));
#18608=CARTESIAN_POINT('Origin',(37.0412526479213,187.739737607024,272.073593133701));
#18609=CARTESIAN_POINT('Origin',(77.1627332513468,100.535558183572,272.073593133701));
#18610=CARTESIAN_POINT('',(-235.81010437183,161.555364540059,239.073593133701));
#18611=CARTESIAN_POINT('',(77.1627332513468,100.535558183572,239.073593133701));
#18612=CARTESIAN_POINT('',(-235.81010437183,161.555364540059,232.073593133701));
#18613=CARTESIAN_POINT('',(-235.81010437183,161.555364540059,272.073593133701));
#18614=CARTESIAN_POINT('Ctrl Pts',(-235.81010437183,161.555364540059,232.073593133701));
#18615=CARTESIAN_POINT('Ctrl Pts',(-233.401640601645,161.085790266491,232.969598917216));
#18616=CARTESIAN_POINT('Ctrl Pts',(-230.521958535878,160.524343326381,234.073593133701));
#18617=CARTESIAN_POINT('Ctrl Pts',(-227.957953056828,160.0244433382,234.073593133701));
#18618=CARTESIAN_POINT('Origin',(-232.939627118345,176.278148255689,276.073593133701));
#18619=CARTESIAN_POINT('',(-217.93964885286,176.303683231751,275.773593133701));
#18620=CARTESIAN_POINT('Origin',(-232.939627118345,176.278148255689,275.773593133701));
#18621=CARTESIAN_POINT('',(-218.23964841817,176.30317253223,276.073593133701));
#18622=CARTESIAN_POINT('',(-218.23964841817,176.30317253223,276.073593133701));
#18623=CARTESIAN_POINT('Origin',(-232.939627118345,176.278148255689,276.073593133701));
#18624=CARTESIAN_POINT('Origin',(-232.939627118345,176.278148255689,230.373593133701));
#18625=CARTESIAN_POINT('',(-217.939648852861,176.303683231751,230.373593133701));
#18626=CARTESIAN_POINT('',(-247.939605383829,176.252613279627,230.373593133701));
#18627=CARTESIAN_POINT('Origin',(-232.939627118345,176.278148255689,230.373593133701));
#18628=CARTESIAN_POINT('Origin',(-232.939627118345,176.278148255689,230.373593133701));
#18629=CARTESIAN_POINT('',(-247.639605818519,176.253123979149,230.073593133701));
#18630=CARTESIAN_POINT('',(-247.939605383829,176.252613279627,230.373593133701));
#18631=CARTESIAN_POINT('Origin',(-232.939627118345,176.278148255689,230.073593133701));
#18632=CARTESIAN_POINT('Origin',(-232.939627118345,176.278148255689,274.073593133701));
#18633=CARTESIAN_POINT('',(-217.93964885286,176.303683231751,274.073593133701));
#18634=CARTESIAN_POINT('Origin',(-232.939627118345,176.278148255689,274.073593133701));
#18635=CARTESIAN_POINT('',(-235.587533185649,191.042585036641,274.073593133701));
#18636=CARTESIAN_POINT('Ctrl Pts',(-235.587533185649,191.042585036641,274.073593133701));
#18637=CARTESIAN_POINT('Ctrl Pts',(-233.172255493539,191.475749440407,273.177587350186));
#18638=CARTESIAN_POINT('Ctrl Pts',(-230.28442635535,191.993662884028,272.073593133701));
#18639=CARTESIAN_POINT('Ctrl Pts',(-227.713166902474,192.45480160587,272.073593133701));
#18640=CARTESIAN_POINT('Origin',(-232.939627118345,176.278148255689,274.073593133701));
#18641=CARTESIAN_POINT('Origin',(-232.939627118345,176.278148255689,232.073593133701));
#18642=CARTESIAN_POINT('',(-217.93964885286,176.303683231751,232.073593133701));
#18643=CARTESIAN_POINT('Origin',(-232.939627118345,176.278148255689,232.073593133701));
#18644=CARTESIAN_POINT('',(-235.587533185649,191.042585036641,232.073593133701));
#18645=CARTESIAN_POINT('Origin',(-232.939627118345,176.278148255689,232.073593133701));
#18646=CARTESIAN_POINT('Ctrl Pts',(-227.713166902474,192.45480160587,234.073593133701));
#18647=CARTESIAN_POINT('Ctrl Pts',(-228.302971253065,192.349024017356,234.073593133701));
#18648=CARTESIAN_POINT('Ctrl Pts',(-228.946265347253,192.233653389927,234.011051403062));
#18649=CARTESIAN_POINT('Ctrl Pts',(-230.220656559869,192.005099583638,233.79592036922));
#18650=CARTESIAN_POINT('Ctrl Pts',(-230.852002282766,191.891871819177,233.644853883273));
#18651=CARTESIAN_POINT('Ctrl Pts',(-232.746921387808,191.552030356226,233.122017490068));
#18652=CARTESIAN_POINT('Ctrl Pts',(-234.297116814936,191.274012851197,232.552304353979));
#18653=CARTESIAN_POINT('Ctrl Pts',(-235.587533185649,191.042585036641,232.073593133701));
#18654=CARTESIAN_POINT('Origin',(43.6251949327106,132.560865708529,272.073593133701));
#18655=CARTESIAN_POINT('',(54.6251789940657,132.579591357641,272.073593133701));
#18656=CARTESIAN_POINT('Origin',(37.0412526479213,187.739737607024,272.073593133701));
#18657=CARTESIAN_POINT('',(45.0412410561795,187.753356260924,272.073593133701));
#18658=CARTESIAN_POINT('Origin',(-232.939627118345,176.278148255689,272.073593133701));
#18659=CARTESIAN_POINT('',(-224.939638710086,176.291766909589,276.073593133701));
#18660=CARTESIAN_POINT('Origin',(-232.939627118345,176.278148255689,276.073593133701));
#18661=CARTESIAN_POINT('',(-224.939638710086,176.291766909589,272.073593133701));
#18662=CARTESIAN_POINT('Origin',(-232.939627118345,176.278148255689,272.073593133701));
#18663=CARTESIAN_POINT('',(-217.93964885286,176.303683231751,272.073593133701));
#18664=CARTESIAN_POINT('',(-235.587533185649,191.042585036641,239.073593133701));
#18665=CARTESIAN_POINT('Origin',(-232.939627118345,176.278148255689,239.073593133701));
#18666=CARTESIAN_POINT('',(-235.587533185649,191.042585036641,272.073593133701));
#18667=CARTESIAN_POINT('Origin',(43.6251949327106,132.560865708529,272.073593133701));
#18668=CARTESIAN_POINT('',(54.6251789940657,132.579591357641,239.073593133701));
#18669=CARTESIAN_POINT('Origin',(43.6251949327106,132.560865708529,239.073593133701));
#18670=CARTESIAN_POINT('',(54.6251789940657,132.579591357641,272.073593133701));
#18671=CARTESIAN_POINT('Origin',(37.0412526479213,187.739737607024,272.073593133701));
#18672=CARTESIAN_POINT('',(45.0412410561795,187.753356260924,239.073593133701));
#18673=CARTESIAN_POINT('Origin',(37.0412526479213,187.739737607024,239.073593133701));
#18674=CARTESIAN_POINT('',(45.0412410561795,187.753356260924,272.073593133701));
#18675=CARTESIAN_POINT('Origin',(-232.939627118345,176.278148255689,272.073593133701));
#18676=CARTESIAN_POINT('',(-224.939638710086,176.291766909589,239.073593133701));
#18677=CARTESIAN_POINT('Origin',(-232.939627118345,176.278148255689,239.073593133701));
#18678=CARTESIAN_POINT('',(-224.939638710086,176.291766909589,230.073593133701));
#18679=CARTESIAN_POINT('',(-224.939638710086,176.291766909589,272.073593133701));
#18680=CARTESIAN_POINT('Origin',(-232.939627118345,176.278148255689,230.073593133701));
#18681=CARTESIAN_POINT('Origin',(-232.939627118345,176.278148255689,272.073593133701));
#18682=CARTESIAN_POINT('',(-217.93964885286,176.303683231751,272.073593133701));
#18683=CARTESIAN_POINT('',(-235.587533185649,191.042585036641,272.073593133701));
#18684=CARTESIAN_POINT('Origin',(76.9784177883129,208.807754437623,239.073593133701));
#18685=CARTESIAN_POINT('',(-175.410387021446,208.378104342469,241.073593133701));
#18686=CARTESIAN_POINT('',(-175.410387021446,208.378104342469,265.073593133701));
#18687=CARTESIAN_POINT('',(-175.410387021446,208.378104342469,239.073593133701));
#18688=CARTESIAN_POINT('',(46.4156250629116,208.755726350194,241.073593133701));
#18689=CARTESIAN_POINT('',(46.4156250629116,208.755726350194,241.073593133701));
#18690=CARTESIAN_POINT('',(46.4156250629116,208.755726350194,265.073593133701));
#18691=CARTESIAN_POINT('',(46.4156250629116,208.755726350194,239.073593133701));
#18692=CARTESIAN_POINT('',(-175.410387021446,208.378104342469,265.073593133701));
#18693=CARTESIAN_POINT('Origin',(31.8750805350466,183.730937259653,272.073593133701));
#18694=CARTESIAN_POINT('',(31.824010582923,213.730893790622,239.073593133701));
#18695=CARTESIAN_POINT('Ctrl Pts',(48.4156221649759,208.759131013669,234.073593133701));
#18696=CARTESIAN_POINT('Ctrl Pts',(47.1896385418122,209.56935461014,234.073593133701));
#18697=CARTESIAN_POINT('Ctrl Pts',(45.8893226556104,210.298387522342,234.266240084391));
#18698=CARTESIAN_POINT('Ctrl Pts',(43.182667391614,211.558385445743,234.877469643646));
#18699=CARTESIAN_POINT('Ctrl Pts',(41.7767242102558,212.088894220586,235.29874407437));
#18700=CARTESIAN_POINT('Ctrl Pts',(37.4929130147176,213.350222803775,236.749321829369));
#18701=CARTESIAN_POINT('Ctrl Pts',(34.5450346732006,213.735525883001,237.962738090941));
#18702=CARTESIAN_POINT('Ctrl Pts',(31.824010582923,213.730893790622,239.073593133701));
#18703=CARTESIAN_POINT('',(31.824010582923,213.730893790622,267.073593133701));
#18704=CARTESIAN_POINT('',(31.824010582923,213.730893790622,272.073593133701));
#18705=CARTESIAN_POINT('Ctrl Pts',(31.8240105829231,213.730893790622,267.073593133701));
#18706=CARTESIAN_POINT('Ctrl Pts',(33.2842831762373,213.733379662604,267.669747787341));
#18707=CARTESIAN_POINT('Ctrl Pts',(34.8844074857718,213.623034356201,268.324081712763));
#18708=CARTESIAN_POINT('Ctrl Pts',(38.067190631896,213.129088570913,269.562579881701));
#18709=CARTESIAN_POINT('Ctrl Pts',(39.6508266059049,212.744886046318,270.143991098496));
#18710=CARTESIAN_POINT('Ctrl Pts',(42.2750677822305,211.898355182682,270.994988064577));
#18711=CARTESIAN_POINT('Ctrl Pts',(43.5675862165289,211.393971522727,271.369518426275));
#18712=CARTESIAN_POINT('Ctrl Pts',(46.0918857841089,210.185438113252,271.910455807107));
#18713=CARTESIAN_POINT('Ctrl Pts',(47.3240128653335,209.480549796096,272.073593133701));
#18714=CARTESIAN_POINT('Ctrl Pts',(48.415622164976,208.759131013669,272.073593133701));
#18715=CARTESIAN_POINT('',(61.4104021126536,188.99066912614,272.073593133701));
#18716=CARTESIAN_POINT('',(46.4135532795135,209.972751416803,239.073593133701));
#18717=CARTESIAN_POINT('',(46.4135532795135,209.972751416803,272.073593133701));
#18718=CARTESIAN_POINT('',(61.4104021126536,188.99066912614,239.073593133701));
#18719=CARTESIAN_POINT('Origin',(31.8750805350466,183.730937259653,239.073593133701));
#18720=CARTESIAN_POINT('',(61.4104021126536,188.99066912614,272.073593133701));
#18721=CARTESIAN_POINT('Origin',(-169.989089387034,205.387328855953,272.073593133701));
#18722=CARTESIAN_POINT('',(-170.002708040934,213.387317264211,239.073593133701));
#18723=CARTESIAN_POINT('',(-170.002708040934,213.387317264211,267.073593133701));
#18724=CARTESIAN_POINT('',(-170.002708040934,213.387317264211,272.073593133701));
#18725=CARTESIAN_POINT('Ctrl Pts',(-170.002708040934,213.387317264211,239.073593133701));
#18726=CARTESIAN_POINT('Ctrl Pts',(-170.753749210153,213.38603874114,238.479842095552));
#18727=CARTESIAN_POINT('Ctrl Pts',(-171.571319487893,213.273469607744,237.832779229032));
#18728=CARTESIAN_POINT('Ctrl Pts',(-173.16290966802,212.777967370924,236.600716776795));
#18729=CARTESIAN_POINT('Ctrl Pts',(-173.937251007441,212.394457262387,236.016364655997));
#18730=CARTESIAN_POINT('Ctrl Pts',(-175.162834807223,211.526126218123,235.150121220116));
#18731=CARTESIAN_POINT('Ctrl Pts',(-175.728422301512,211.014823745933,234.774113289777));
#18732=CARTESIAN_POINT('Ctrl Pts',(-176.707530587388,209.799946719515,234.234922296038));
#18733=CARTESIAN_POINT('Ctrl Pts',(-177.120418024857,209.095040075002,234.073593133701));
#18734=CARTESIAN_POINT('Ctrl Pts',(-177.41038412351,208.374699678994,234.073593133701));
#18735=CARTESIAN_POINT('',(-177.989077795293,205.373710202053,239.073593133701));
#18736=CARTESIAN_POINT('',(-177.989077795293,205.373710202053,272.073593133701));
#18737=CARTESIAN_POINT('',(-175.415302813384,211.265781701023,239.073593133701));
#18738=CARTESIAN_POINT('Origin',(-169.989089387034,205.387328855953,239.073593133701));
#18739=CARTESIAN_POINT('',(-175.415302813384,211.265781701023,272.073593133701));
#18740=CARTESIAN_POINT('',(-177.989077795293,205.373710202053,272.073593133701));
#18741=CARTESIAN_POINT('Ctrl Pts',(-177.41038412351,208.374699678994,272.073593133701));
#18742=CARTESIAN_POINT('Ctrl Pts',(-177.148926429536,209.024218845859,272.073593133701));
#18743=CARTESIAN_POINT('Ctrl Pts',(-176.783223638279,209.670726923257,271.94133193636));
#18744=CARTESIAN_POINT('Ctrl Pts',(-175.919217012443,210.804093658125,271.487456150798));
#18745=CARTESIAN_POINT('Ctrl Pts',(-175.421532019632,211.292236733482,271.167874220512));
#18746=CARTESIAN_POINT('Ctrl Pts',(-174.223592818156,212.235297258746,270.34369109411));
#18747=CARTESIAN_POINT('Ctrl Pts',(-173.398721571726,212.680063455512,269.726299154576));
#18748=CARTESIAN_POINT('Ctrl Pts',(-171.69360491859,213.25525034828,268.411275830787));
#18749=CARTESIAN_POINT('Ctrl Pts',(-170.813019784585,213.385937842814,267.714201743102));
#18750=CARTESIAN_POINT('Ctrl Pts',(-170.002708040934,213.387317264211,267.073593133701));
#18751=CARTESIAN_POINT('Origin',(-177.982268468343,201.373715997924,272.073593133701));
#18752=CARTESIAN_POINT('',(-177.982268468343,201.373715997924,272.073593133701));
#18753=CARTESIAN_POINT('Origin',(56.9969630433931,213.773746568613,272.073593133701));
#18754=CARTESIAN_POINT('',(70.7697436798221,136.43453699661,239.073593133701));
#18755=CARTESIAN_POINT('',(56.9969630433931,213.773746568613,239.073593133701));
#18756=CARTESIAN_POINT('',(70.7697436798221,136.43453699661,272.073593133701));
#18757=CARTESIAN_POINT('Origin',(-235.587533185649,191.042585036641,272.073593133701));
#18758=CARTESIAN_POINT('',(-177.982268468343,201.373715997924,239.073593133701));
#18759=CARTESIAN_POINT('',(-235.587533185649,191.042585036641,239.073593133701));
#18760=CARTESIAN_POINT('',(-177.982268468343,201.373715997924,272.073593133701));
#18761=CARTESIAN_POINT('Origin',(56.9969630433931,213.773746568613,272.073593133701));
#18762=CARTESIAN_POINT('',(70.7697436798221,136.43453699661,272.073593133701));
#18763=CARTESIAN_POINT('Origin',(-178.002696449192,213.373698610312,272.073593133701));
#18764=CARTESIAN_POINT('',(-178.002696449192,213.373698610312,239.073593133701));
#18765=CARTESIAN_POINT('',(31.824010582923,213.730893790622,267.073593133701));
#18766=CARTESIAN_POINT('Origin',(-177.982268468343,201.373715997924,272.073593133701));
#18767=CARTESIAN_POINT('',(-177.982268468343,201.373715997924,239.073593133701));
#18768=CARTESIAN_POINT('Origin',(-235.587533185649,191.042585036641,272.073593133701));
#18769=CARTESIAN_POINT('Origin',(76.9784177883129,208.807754437623,239.073593133701));
#18770=CARTESIAN_POINT('Origin',(46.1569756984829,132.05142710787,239.073593133701));
#18771=CARTESIAN_POINT('',(46.4190297263865,206.75572924813,239.073593133701));
#18772=CARTESIAN_POINT('',(46.5887585805977,107.052125922394,239.073593133701));
#18773=CARTESIAN_POINT('',(-175.406982357971,206.378107240404,239.073593133701));
#18774=CARTESIAN_POINT('',(-175.406982357971,206.378107240404,239.073593133701));
#18775=CARTESIAN_POINT('',(-175.23725350376,106.674503914668,239.073593133701));
#18776=CARTESIAN_POINT('Origin',(-232.939627118345,176.278148255689,276.073593133701));
#18777=CARTESIAN_POINT('Origin',(-232.939627118345,176.278148255689,230.073593133701));
#18778=CARTESIAN_POINT('Origin',(46.1569756984829,132.05142710787,272.073593133701));
#18779=CARTESIAN_POINT('Origin',(46.1569756984829,132.05142710787,272.073593133701));
#18780=CARTESIAN_POINT('Origin',(-175.23725350376,106.674503914668,267.073593133701));
#18781=CARTESIAN_POINT('Origin',(-175.406982357971,206.378107240404,241.073593133701));
#18782=CARTESIAN_POINT('Origin',(-175.406982357971,206.378107240404,265.073593133701));
#18783=CARTESIAN_POINT('Origin',(46.5887585805977,107.052125922394,267.073593133701));
#18784=CARTESIAN_POINT('Origin',(46.4190297263865,206.75572924813,265.073593133701));
#18785=CARTESIAN_POINT('Origin',(46.4190297263865,206.75572924813,241.073593133701));
#18786=CARTESIAN_POINT('Origin',(-177.994184790505,208.37370585515,239.073593133701));
#18787=CARTESIAN_POINT('Origin',(-232.99410509728,208.28007760959,267.073593133701));
#18788=CARTESIAN_POINT('Origin',(76.9818224517878,206.807757335558,241.073593133701));
#18789=CARTESIAN_POINT('Origin',(76.9818224517878,206.807757335558,265.073593133701));
#27753=UNCERTAINTY_MEASURE_WITH_UNIT(LENGTH_MEASURE(0.01),#27808,
'DISTANCE_ACCURACY_VALUE',
'Maximum model space distance between geometric entities at asserted c
onnectivities');
#27778=UNCERTAINTY_MEASURE_WITH_UNIT(LENGTH_MEASURE(0.01),#27808,
'DISTANCE_ACCURACY_VALUE',
'Maximum model space distance between geometric entities at asserted c
onnectivities');
#27782=(
GEOMETRIC_REPRESENTATION_CONTEXT(3)
GLOBAL_UNCERTAINTY_ASSIGNED_CONTEXT((#27753))
GLOBAL_UNIT_ASSIGNED_CONTEXT((#27808,#27810,#27811))
REPRESENTATION_CONTEXT('','3D')
);
#27807=(
GEOMETRIC_REPRESENTATION_CONTEXT(3)
GLOBAL_UNCERTAINTY_ASSIGNED_CONTEXT((#27778))
GLOBAL_UNIT_ASSIGNED_CONTEXT((#27808,#27810,#27811))
REPRESENTATION_CONTEXT('','3D')
);
#27808=(
LENGTH_UNIT()
NAMED_UNIT(*)
SI_UNIT(.MILLI.,.METRE.)
);
#27810=(
NAMED_UNIT(*)
PLANE_ANGLE_UNIT()
SI_UNIT($,.RADIAN.)
);
#27811=(
NAMED_UNIT(*)
SI_UNIT($,.STERADIAN.)
SOLID_ANGLE_UNIT()
);
#27815=SHAPE_DEFINITION_REPRESENTATION(#27843,#27902);
#27843=PRODUCT_DEFINITION_SHAPE('',$,#27931);
#27902=SHAPE_REPRESENTATION('',(#12653),#27782);
#27927=PRODUCT_DEFINITION_CONTEXT('part definition',#28013,'design');
#27931=PRODUCT_DEFINITION('Lifting Arm','Lifting Arm',#27959,#27927);
#27959=PRODUCT_DEFINITION_FORMATION('',$,#28018);
#28013=APPLICATION_CONTEXT('Managed model based 3d engineering');
#28014=PRODUCT_CONTEXT('part definition',#28013,'mechanical');
#28018=PRODUCT('Lifting Arm','Lifting Arm',$,(#28014));
#28064=COLOUR_RGB('Sky Blue',0.24,0.69,0.87);
#28065=FILL_AREA_STYLE_COLOUR('',#28064);
#28066=FILL_AREA_STYLE('',(#28065));
#28067=SURFACE_STYLE_FILL_AREA(#28066);
#28068=SURFACE_SIDE_STYLE('',(#28067));
#28069=SURFACE_STYLE_USAGE(.BOTH.,#28068);
#28070=PRESENTATION_STYLE_ASSIGNMENT((#28069));
ENDSEC;
END-ISO-10303-21;
